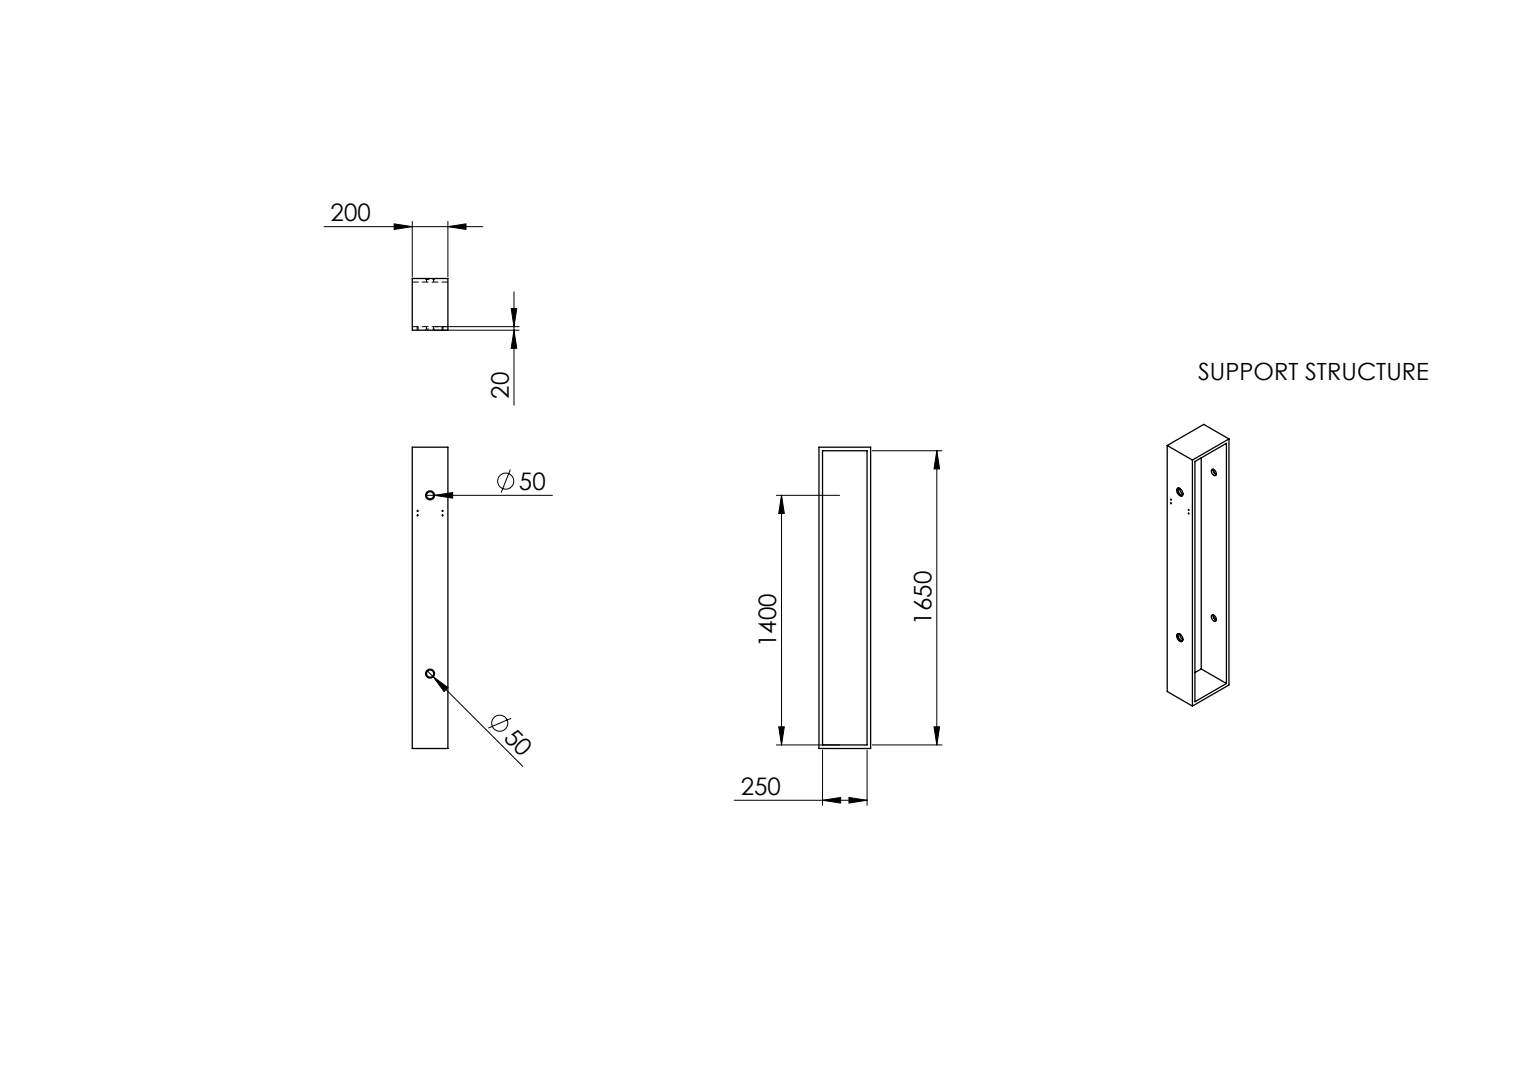
ISO-10303-21;
HEADER;
FILE_DESCRIPTION (('STEP AP214'),
    '1' );
FILE_NAME ('support structure.step',
    '2026-10-31T03:46:07',
    ( '' ),
    ( '' ),
    'SwSTEP 2.0',
    'SolidWorks 2026',
    '' );
FILE_SCHEMA (( 'AUTOMOTIVE_DESIGN' ));
ENDSEC;

DATA;
#3=VECTOR ( 'NONE', #6324, 1000.000000000000000 ) ;
#6=CARTESIAN_POINT ( 'NONE',  ( 18.83467029480910071, -16.52066876451827326, 145.0000119999999697 ) ) ;
#19=EDGE_CURVE ( 'NONE', #8380, #2021, #17168, .T. ) ;
#27=DIRECTION ( 'NONE',  ( 0.000000000000000000, 1.177509268541832635E-16, -1.000000000000000000 ) ) ;
#28=CARTESIAN_POINT ( 'NONE',  ( 15.24974479720505549, -1019.877690639539310, 145.0000119999999697 ) ) ;
#41=ORIENTED_EDGE ( 'NONE', *, *, #15976, .F. ) ;
#54=EDGE_LOOP ( 'NONE', ( #6384, #11170, #16002, #7000 ) ) ;
#58=DIRECTION ( 'NONE',  ( -1.000000000000000000, 0.000000000000000000, 0.000000000000000000 ) ) ;
#77=CARTESIAN_POINT ( 'NONE',  ( -69.99999999999997158, -87.33333333333338544, 145.0000000000000000 ) ) ;
#79=ORIENTED_EDGE ( 'NONE', *, *, #18426, .F. ) ;
#86=DIRECTION ( 'NONE',  ( 1.000000000000000000, 0.000000000000000000, 0.000000000000000000 ) ) ;
#96=CARTESIAN_POINT ( 'NONE',  ( 0.000000000000000000, -1000.000000000000000, 138.9999999999999716 ) ) ;
#102=CARTESIAN_POINT ( 'NONE',  ( 100.0000000000000000, 249.9999999999999716, 125.0000000000000284 ) ) ;
#108=LINE ( 'NONE', #2015, #19648 ) ;
#115=CARTESIAN_POINT ( 'NONE',  ( -11.07878015919984982, -22.47082401081930669, 145.0000119999999697 ) ) ;
#165=CIRCLE ( 'NONE', #9426, 5.249999999999949374 ) ;
#175=ORIENTED_EDGE ( 'NONE', *, *, #23587, .F. ) ;
#179=EDGE_CURVE ( 'NONE', #21239, #21516, #2397, .T. ) ;
#193=DIRECTION ( 'NONE',  ( 0.000000000000000000, 1.177509268541832635E-16, -1.000000000000000000 ) ) ;
#207=AXIS2_PLACEMENT_3D ( 'NONE', #19783, #10642, #8811 ) ;
#218=VERTEX_POINT ( 'NONE', #2274 ) ;
#224=DIRECTION ( 'NONE',  ( 0.000000000000000000, -1.000000000000000000, -1.177509268541832635E-16 ) ) ;
#245=EDGE_LOOP ( 'NONE', ( #12750, #13760, #3479, #23001 ) ) ;
#247=CYLINDRICAL_SURFACE ( 'NONE', #10836, 20.00000000000000000 ) ;
#257=ORIENTED_EDGE ( 'NONE', *, *, #4493, .F. ) ;
#312=DIRECTION ( 'NONE',  ( 0.000000000000000000, -1.000000000000000000, 0.000000000000000000 ) ) ;
#342=CARTESIAN_POINT ( 'NONE',  ( -24.99999999999998224, -1000.000000000000000, -145.0000119999999697 ) ) ;
#356=CARTESIAN_POINT ( 'NONE',  ( 21.69578997558840072, -12.52876685377503740, 145.0000119999999697 ) ) ;
#358=ADVANCED_FACE ( 'NONE', ( #20999 ), #19173, .F. ) ;
#362=PRODUCT_DEFINITION_CONTEXT ( 'detailed design', #17104, 'design' ) ;
#375=DIRECTION ( 'NONE',  ( -0.000000000000000000, 1.000000000000000000, -0.000000000000000000 ) ) ;
#385=CARTESIAN_POINT ( 'NONE',  ( 24.83884780301425721, -996.7275481119215783, 145.0000119999999981 ) ) ;
#391=ORIENTED_EDGE ( 'NONE', *, *, #9476, .F. ) ;
#411=ORIENTED_EDGE ( 'NONE', *, *, #12338, .T. ) ;
#419=DIRECTION ( 'NONE',  ( 0.000000000000000000, 1.177509268541832635E-16, -1.000000000000000000 ) ) ;
#431=EDGE_CURVE ( 'NONE', #23382, #2113, #16801, .T. ) ;
#434=LINE ( 'NONE', #15168, #15820 ) ;
#446=DIRECTION ( 'NONE',  ( 0.000000000000000000, -1.177509268541832635E-16, 1.000000000000000000 ) ) ;
#448=CARTESIAN_POINT ( 'NONE',  ( 70.00000000000000000, -87.33333333333332860, 124.9999999999999858 ) ) ;
#463=ADVANCED_FACE ( 'NONE', ( #11105 ), #20128, .F. ) ;
#476=DIRECTION ( 'NONE',  ( -0.000000000000000000, -0.000000000000000000, 1.000000000000000000 ) ) ;
#485=CARTESIAN_POINT ( 'NONE',  ( -45.00000000000000000, 272.9999999999999432, 0.000000000000000000 ) ) ;
#490=EDGE_CURVE ( 'NONE', #8328, #14713, #20594, .T. ) ;
#496=CARTESIAN_POINT ( 'NONE',  ( -24.99999999999998224, -1000.000000000000000, -145.0000060000000417 ) ) ;
#527=LINE ( 'NONE', #18858, #1845 ) ;
#529=ORIENTED_EDGE ( 'NONE', *, *, #11440, .F. ) ;
#546=CYLINDRICAL_SURFACE ( 'NONE', #5912, 20.00000000000000000 ) ;
#562=FACE_BOUND ( 'NONE', #6176, .T. ) ;
#563=DIRECTION ( 'NONE',  ( 0.000000000000000000, 0.000000000000000000, 1.000000000000000000 ) ) ;
#567=FACE_OUTER_BOUND ( 'NONE', #20459, .T. ) ;
#570=FACE_OUTER_BOUND ( 'NONE', #6214, .T. ) ;
#574=CARTESIAN_POINT ( 'NONE',  ( -69.99999999999997158, -112.6666666666667140, 124.9999999999999858 ) ) ;
#575=DIRECTION ( 'NONE',  ( 0.000000000000000000, 1.000000000000000000, 0.000000000000000000 ) ) ;
#576=ORIENTED_EDGE ( 'NONE', *, *, #2075, .T. ) ;
#589=CLOSED_SHELL ( 'NONE', ( #11368, #788, #23385, #20795, #2609, #21444, #6790, #9900, #8687, #7105, #11204, #10218, #16290, #19058, #463, #16239, #358, #10479, #18110, #9024, #1914, #5319, #16488, #1601, #20906, #2345, #19700, #11952, #5464, #626, #8870, #13898, #20498, #5716, #16281, #4561, #17901, #4387, #5710, #23652, #11628, #12501, #17871, #17586, #23607, #23039, #14935, #17741, #20750, #1436 ) ) ;
#612=CARTESIAN_POINT ( 'NONE',  ( -3.267023609986814847, -1024.839877336693462, -145.0000000000001421 ) ) ;
#615=CARTESIAN_POINT ( 'NONE',  ( 18.83467029480909005, -983.4793312354817090, 145.0000119999999697 ) ) ;
#626=ADVANCED_FACE ( 'NONE', ( #13405, #570 ), #13541, .T. ) ;
#637=DIRECTION ( 'NONE',  ( -0.000000000000000000, -0.000000000000000000, 1.000000000000000000 ) ) ;
#642=AXIS2_PLACEMENT_3D ( 'NONE', #1473, #5465, #8869 ) ;
#654=DIRECTION ( 'NONE',  ( 1.000000000000000000, 0.000000000000000000, 0.000000000000000000 ) ) ;
#657=DIRECTION ( 'NONE',  ( 0.000000000000000000, 1.177509268541832635E-16, -1.000000000000000000 ) ) ;
#665=ORIENTED_EDGE ( 'NONE', *, *, #13392, .T. ) ;
#670=LINE ( 'NONE', #6231, #14453 ) ;
#675=FACE_BOUND ( 'NONE', #20400, .T. ) ;
#691=DIRECTION ( 'NONE',  ( 0.000000000000000000, -1.177509268541832635E-16, 1.000000000000000000 ) ) ;
#702=CARTESIAN_POINT ( 'NONE',  ( -45.24999999999994316, 100.0000000000000000, -125.0000000000000000 ) ) ;
#710=CARTESIAN_POINT ( 'NONE',  ( -24.99999999999998224, -1000.000000000000000, 145.0000119999999697 ) ) ;
#719=AXIS2_PLACEMENT_3D ( 'NONE', #14243, #1403, #19754 ) ;
#735=STYLED_ITEM('',(#23934),#20017);
#755=CARTESIAN_POINT ( 'NONE',  ( -16.51661848988935688, -981.1612097654584659, -145.0000000000001137 ) ) ;
#777=CARTESIAN_POINT ( 'NONE',  ( 67.35000000000002274, -112.6666666666666714, 148.0000000000000000 ) ) ;
#788=ADVANCED_FACE ( 'NONE', ( #20967 ), #6715, .F. ) ;
#791=CARTESIAN_POINT ( 'NONE',  ( -15.25452100743371275, 19.87444003246448077, -145.0000000000000000 ) ) ;
#798=CYLINDRICAL_SURFACE ( 'NONE', #13137, 20.00000000000000000 ) ;
#815=DIRECTION ( 'NONE',  ( -1.000000000000000000, -0.000000000000000000, -0.000000000000000000 ) ) ;
#853=CARTESIAN_POINT ( 'NONE',  ( 16.51667796972429514, -18.83873075115305440, -145.0000000000000000 ) ) ;
#864=CARTESIAN_POINT ( 'NONE',  ( -24.19933745276217252, -993.5122599704404820, -145.0000000000001137 ) ) ;
#883=FACE_BOUND ( 'NONE', #18234, .T. ) ;
#888=CYLINDRICAL_SURFACE ( 'NONE', #2282, 20.00000000000000000 ) ;
#891=CARTESIAN_POINT ( 'NONE',  ( -21.69892645963121325, 12.52401366518118841, -145.0000000000000000 ) ) ;
#903=ORIENTED_EDGE ( 'NONE', *, *, #3665, .F. ) ;
#916=FACE_BOUND ( 'NONE', #6482, .T. ) ;
#917=DIRECTION ( 'NONE',  ( 1.000000000000000000, 0.000000000000000000, 0.000000000000000000 ) ) ;
#926=CARTESIAN_POINT ( 'NONE',  ( 0.000000000000000000, 0.000000000000000000, 138.9999999999999716 ) ) ;
#930=CIRCLE ( 'NONE', #16749, 5.249999999999949374 ) ;
#940=EDGE_CURVE ( 'NONE', #17429, #3770, #2550, .T. ) ;
#948=CYLINDRICAL_SURFACE ( 'NONE', #18630, 2.649999999999985700 ) ;
#954=DIRECTION ( 'NONE',  ( -1.000000000000000000, -0.000000000000000000, -0.000000000000000000 ) ) ;
#965=CARTESIAN_POINT ( 'NONE',  ( -23.72540896994113524, -8.050072860292576848, -145.0000000000000000 ) ) ;
#975=CARTESIAN_POINT ( 'NONE',  ( -1.642023387942652235, -975.0000492607058504, -145.0000000000001421 ) ) ;
#981=SURFACE_STYLE_USAGE ( .BOTH. , #17532 ) ;
#997=B_SPLINE_CURVE_WITH_KNOTS ( 'NONE', 3,
 ( #16561, #14521, #9199, #21855, #11385, #5449, #16437, #14640, #23787, #12745, #3867, #5814, #18479, #16679, #5326, #16789, #14756, #7484, #18699, #20277, #9325, #7604, #12857, #28, #20057, #10914, #18236, #9077, #14997, #13218, #20519, #22087, #3732, #7245 ),
 .UNSPECIFIED., .F., .F.,
 ( 4, 2, 2, 2, 2, 2, 2, 2, 2, 2, 2, 2, 2, 2, 2, 2, 4 ),
 ( 0.5000000000000000000, 0.5312500000000000000, 0.5625000000000000000, 0.5937500000000000000, 0.6250000000000000000, 0.6562500000000000000, 0.6875000000000000000, 0.7187500000000000000, 0.7500000000000000000, 0.7812500000000000000, 0.8125000000000000000, 0.8437500000000000000, 0.8750000000000000000, 0.9062500000000000000, 0.9375000000000000000, 0.9687500000000000000, 1.000000000000000000 ),
 .UNSPECIFIED. ) ;
#1003=DIRECTION ( 'NONE',  ( 0.000000000000000000, 1.000000000000000000, 0.000000000000000000 ) ) ;
#1007=CARTESIAN_POINT ( 'NONE',  ( 6.487740029101478179, 24.19933745276211212, -145.0000000000000000 ) ) ;
#1022=CYLINDRICAL_SURFACE ( 'NONE', #9203, 25.00000000000000000 ) ;
#1068=FACE_OUTER_BOUND ( 'NONE', #19426, .T. ) ;
#1088=CARTESIAN_POINT ( 'NONE',  ( 12.52399064345484980, -21.69904058272398117, -145.0000000000000000 ) ) ;
#1106=ORIENTED_EDGE ( 'NONE', *, *, #5078, .F. ) ;
#1142=CIRCLE ( 'NONE', #20035, 2.649999999999999467 ) ;
#1161=STYLED_ITEM ( 'NONE', ( #8363 ), #19351 ) ;
#1173=EDGE_LOOP ( 'NONE', ( #15595, #19148, #21434, #576 ) ) ;
#1179=CYLINDRICAL_SURFACE ( 'NONE', #16892, 5.249999999999973355 ) ;
#1187=CARTESIAN_POINT ( 'NONE',  ( 67.35000000000002274, -87.33333333333332860, 124.9999999999999858 ) ) ;
#1198=LINE ( 'NONE', #13923, #16019 ) ;
#1200=ORIENTED_EDGE ( 'NONE', *, *, #4425, .F. ) ;
#1202=DIRECTION ( 'NONE',  ( 1.000000000000000000, 0.000000000000000000, 0.000000000000000000 ) ) ;
#1254=ORIENTED_EDGE ( 'NONE', *, *, #16181, .T. ) ;
#1279=CARTESIAN_POINT ( 'NONE',  ( 45.24999999999994316, 100.0000000000000000, 150.2000000000009550 ) ) ;
#1288=CARTESIAN_POINT ( 'NONE',  ( -20.00000000000000000, 2.449293598294706513E-15, -125.0000000000000000 ) ) ;
#1294=CARTESIAN_POINT ( 'NONE',  ( -20.00000000000000000, -1000.000000000000000, 124.9999999999998579 ) ) ;
#1302=DIRECTION ( 'NONE',  ( 0.000000000000000000, 0.000000000000000000, -1.000000000000000000 ) ) ;
#1314=VERTEX_POINT ( 'NONE', #2400 ) ;
#1326=DIRECTION ( 'NONE',  ( 0.000000000000000000, 1.177509268541832635E-16, -1.000000000000000000 ) ) ;
#1339=CYLINDRICAL_SURFACE ( 'NONE', #13540, 24.99999999999998224 ) ;
#1390=DIRECTION ( 'NONE',  ( 0.000000000000000000, 1.177509268541832635E-16, -1.000000000000000000 ) ) ;
#1394=DIRECTION ( 'NONE',  ( -0.000000000000000000, -0.000000000000000000, 1.000000000000000000 ) ) ;
#1403=DIRECTION ( 'NONE',  ( -0.000000000000000000, -1.177509268541832635E-16, 1.000000000000000000 ) ) ;
#1436=ADVANCED_FACE ( 'NONE', ( #13210 ), #20510, .F. ) ;
#1454=DIRECTION ( 'NONE',  ( -1.000000000000000000, 0.000000000000000000, 0.000000000000000000 ) ) ;
#1466=ORIENTED_EDGE ( 'NONE', *, *, #21900, .T. ) ;
#1472=EDGE_CURVE ( 'NONE', #15247, #5237, #1198, .T. ) ;
#1473=CARTESIAN_POINT ( 'NONE',  ( -40.00000000000000000, 100.0000000000000000, 145.0000000000000000 ) ) ;
#1487=VERTEX_POINT ( 'NONE', #8213 ) ;
#1500=VECTOR ( 'NONE', #17474, 1000.000000000000000 ) ;
#1504=CIRCLE ( 'NONE', #2664, 5.249999999999949374 ) ;
#1521=VECTOR ( 'NONE', #15755, 1000.000000000000000 ) ;
#1535=CARTESIAN_POINT ( 'NONE',  ( 6.482064212728078090, 24.20041621714725721, 145.0000119999999697 ) ) ;
#1558=DIRECTION ( 'NONE',  ( 0.000000000000000000, -1.110223024625156540E-16, 1.000000000000000000 ) ) ;
#1572=CARTESIAN_POINT ( 'NONE',  ( 6.482064212728086972, -24.20041621714725011, 145.0000119999999697 ) ) ;
#1578=EDGE_LOOP ( 'NONE', ( #14590, #13725 ) ) ;
#1586=EDGE_CURVE ( 'NONE', #12471, #4961, #8307, .T. ) ;
#1597=ORIENTED_EDGE ( 'NONE', *, *, #13231, .F. ) ;
#1601=ADVANCED_FACE ( 'NONE', ( #9043 ), #3478, .F. ) ;
#1624=CIRCLE ( 'NONE', #13627, 2.649999999999985700 ) ;
#1628=ORIENTED_EDGE ( 'NONE', *, *, #5078, .T. ) ;
#1650=CARTESIAN_POINT ( 'NONE',  ( 0.000000000000000000, 1.865214261513747767E-15, 145.0000119999999697 ) ) ;
#1656=ORIENTED_EDGE ( 'NONE', *, *, #2894, .T. ) ;
#1668=ORIENTED_EDGE ( 'NONE', *, *, #13168, .T. ) ;
#1687=PRODUCT ( 'support structure', 'support structure', '', ( #5653 ) ) ;
#1700=ORIENTED_EDGE ( 'NONE', *, *, #10708, .F. ) ;
#1705=ORIENTED_EDGE ( 'NONE', *, *, #18577, .F. ) ;
#1736=DIRECTION ( 'NONE',  ( -0.000000000000000000, -0.000000000000000000, 1.000000000000000000 ) ) ;
#1788=CARTESIAN_POINT ( 'NONE',  ( -12.52876685377503385, -21.69578997558839717, 145.0000119999999981 ) ) ;
#1809=DIRECTION ( 'NONE',  ( 0.000000000000000000, 0.000000000000000000, 1.000000000000000000 ) ) ;
#1811=LINE ( 'NONE', #9206, #10408 ) ;
#1823=FACE_OUTER_BOUND ( 'NONE', #12229, .T. ) ;
#1825=EDGE_CURVE ( 'NONE', #13236, #17386, #21895, .T. ) ;
#1845=VECTOR ( 'NONE', #954, 1000.000000000000000 ) ;
#1872=FACE_OUTER_BOUND ( 'NONE', #23417, .T. ) ;
#1889=EDGE_LOOP ( 'NONE', ( #14035, #13919, #9509, #20790 ) ) ;
#1907=DIRECTION ( 'NONE',  ( -0.000000000000000000, -0.000000000000000000, 1.000000000000000000 ) ) ;
#1912=ORIENTED_EDGE ( 'NONE', *, *, #7800, .F. ) ;
#1914=ADVANCED_FACE ( 'NONE', ( #17471, #916 ), #21219, .T. ) ;
#1956=VERTEX_POINT ( 'NONE', #10856 ) ;
#1957=DIRECTION ( 'NONE',  ( -0.000000000000000000, -0.000000000000000000, 1.000000000000000000 ) ) ;
#1967=DIRECTION ( 'NONE',  ( 0.000000000000000000, 1.000000000000000000, 0.000000000000000000 ) ) ;
#1991=DIRECTION ( 'NONE',  ( -0.000000000000000000, -0.000000000000000000, 1.000000000000000000 ) ) ;
#2002=EDGE_CURVE ( 'NONE', #18582, #6504, #3774, .T. ) ;
#2006=ORIENTED_EDGE ( 'NONE', *, *, #20259, .F. ) ;
#2015=CARTESIAN_POINT ( 'NONE',  ( 100.0000000000000000, 249.9999999999999716, 125.0000000000000284 ) ) ;
#2019=CARTESIAN_POINT ( 'NONE',  ( -40.00000000000000000, 100.0000000000000000, 125.0000000000000000 ) ) ;
#2020=EDGE_LOOP ( 'NONE', ( #17265, #10424, #23573, #20503 ) ) ;
#2021=VERTEX_POINT ( 'NONE', #18282 ) ;
#2023=EDGE_CURVE ( 'NONE', #16783, #7859, #14353, .T. ) ;
#2043=DIRECTION ( 'NONE',  ( -0.000000000000000000, -0.000000000000000000, 1.000000000000000000 ) ) ;
#2050=( NAMED_UNIT ( * ) SI_UNIT ( $, .STERADIAN. ) SOLID_ANGLE_UNIT ( ) );
#2061=EDGE_CURVE ( 'NONE', #23382, #13229, #21904, .T. ) ;
#2067=DIRECTION ( 'NONE',  ( 1.000000000000000000, 0.000000000000000000, 0.000000000000000000 ) ) ;
#2069=VERTEX_POINT ( 'NONE', #18627 ) ;
#2075=EDGE_CURVE ( 'NONE', #21835, #17715, #16831, .T. ) ;
#2082=CARTESIAN_POINT ( 'NONE',  ( 24.99999999999998224, -1000.000000000000000, 138.9999999999999716 ) ) ;
#2096=CARTESIAN_POINT ( 'NONE',  ( -6.482064212728105623, -975.7995837828526646, 145.0000119999999697 ) ) ;
#2101=EDGE_CURVE ( 'NONE', #2069, #12336, #14538, .T. ) ;
#2113=VERTEX_POINT ( 'NONE', #5610 ) ;
#2118=VERTEX_POINT ( 'NONE', #22257 ) ;
#2120=CYLINDRICAL_SURFACE ( 'NONE', #2712, 20.00000000000000000 ) ;
#2139=ORIENTED_EDGE ( 'NONE', *, *, #12338, .F. ) ;
#2148=DIRECTION ( 'NONE',  ( -0.000000000000000000, 1.000000000000000000, -0.000000000000000000 ) ) ;
#2151=AXIS2_PLACEMENT_3D ( 'NONE', #13145, #20452, #18988 ) ;
#2183=AXIS2_PLACEMENT_3D ( 'NONE', #6288, #21018, #15246 ) ;
#2192=DIRECTION ( 'NONE',  ( 0.000000000000000000, 1.177509268541832635E-16, -1.000000000000000000 ) ) ;
#2214=CARTESIAN_POINT ( 'NONE',  ( -3.272451888078324433, -975.1611521969856540, 145.0000119999999697 ) ) ;
#2232=AXIS2_PLACEMENT_3D ( 'NONE', #15906, #3082, #23243 ) ;
#2260=ORIENTED_EDGE ( 'NONE', *, *, #16101, .T. ) ;
#2263=AXIS2_PLACEMENT_3D ( 'NONE', #3156, #11909, #19217 ) ;
#2270=EDGE_CURVE ( 'NONE', #15596, #21835, #19465, .T. ) ;
#2274=CARTESIAN_POINT ( 'NONE',  ( -25.00000000000000000, 1.865214261513747767E-15, -138.9999999999999716 ) ) ;
#2282=AXIS2_PLACEMENT_3D ( 'NONE', #9976, #11933, #2927 ) ;
#2284=CARTESIAN_POINT ( 'NONE',  ( 72.64999999999999147, -87.33333333333332860, 145.0000000000000000 ) ) ;
#2290=CARTESIAN_POINT ( 'NONE',  ( -34.75000000000005684, 100.0000000000000000, -125.0000000000000000 ) ) ;
#2324=CARTESIAN_POINT ( 'NONE',  ( -24.99999999999998224, -1000.000000000000000, -145.0000060000000417 ) ) ;
#2326=VECTOR ( 'NONE', #14074, 1000.000000000000000 ) ;
#2332=ORIENTED_EDGE ( 'NONE', *, *, #9667, .F. ) ;
#2335=CARTESIAN_POINT ( 'NONE',  ( 45.24999999999994316, 100.0000000000000000, 125.0000000000000000 ) ) ;
#2340=VERTEX_POINT ( 'NONE', #17443 ) ;
#2345=ADVANCED_FACE ( 'NONE', ( #883, #8262, #2577 ), #9970, .T. ) ;
#2367=ORIENTED_EDGE ( 'NONE', *, *, #2518, .F. ) ;
#2393=EDGE_LOOP ( 'NONE', ( #11641, #12163, #21345, #5733 ) ) ;
#2397=LINE ( 'NONE', #6023, #2469 ) ;
#2400=CARTESIAN_POINT ( 'NONE',  ( -45.24999999999994316, 100.0000000000000000, 125.0000000000000000 ) ) ;
#2410=CARTESIAN_POINT ( 'NONE',  ( -15.25457574233255365, -1019.874521950566759, -145.0000000000001137 ) ) ;
#2430=AXIS2_PLACEMENT_3D ( 'NONE', #2688, #637, #10084 ) ;
#2454=LINE ( 'NONE', #4392, #6464 ) ;
#2467=CARTESIAN_POINT ( 'NONE',  ( -19.87455415549606741, 15.25449798579914251, -145.0000000000000000 ) ) ;
#2469=VECTOR ( 'NONE', #9783, 1000.000000000000000 ) ;
#2472=EDGE_CURVE ( 'NONE', #22877, #18582, #8983, .T. ) ;
#2482=FACE_BOUND ( 'NONE', #3832, .T. ) ;
#2491=DIRECTION ( 'NONE',  ( 1.000000000000000000, 0.000000000000000000, -0.000000000000000000 ) ) ;
#2518=EDGE_CURVE ( 'NONE', #12660, #5442, #23460, .T. ) ;
#2524=ORIENTED_EDGE ( 'NONE', *, *, #15478, .T. ) ;
#2525=CARTESIAN_POINT ( 'NONE',  ( 100.0000000000000000, 270.0000000000000000, -144.9999999999999716 ) ) ;
#2532=AXIS2_PLACEMENT_3D ( 'NONE', #17832, #23249, #10011 ) ;
#2538=CARTESIAN_POINT ( 'NONE',  ( -34.75000000000005684, 100.0000000000000000, -145.0000000000000284 ) ) ;
#2550=LINE ( 'NONE', #13707, #11792 ) ;
#2574=DIRECTION ( 'NONE',  ( 0.000000000000000000, 0.000000000000000000, 1.000000000000000000 ) ) ;
#2577=FACE_OUTER_BOUND ( 'NONE', #18376, .T. ) ;
#2580=FACE_OUTER_BOUND ( 'NONE', #2393, .T. ) ;
#2582=FACE_OUTER_BOUND ( 'NONE', #245, .T. ) ;
#2587=CARTESIAN_POINT ( 'NONE',  ( -100.0000000000000000, -1420.000000000000000, -145.0000000000001705 ) ) ;
#2609=ADVANCED_FACE ( 'NONE', ( #11298 ), #16589, .F. ) ;
#2632=AXIS2_PLACEMENT_3D ( 'NONE', #12238, #7885, #20671 ) ;
#2664=AXIS2_PLACEMENT_3D ( 'NONE', #12447, #16140, #4785 ) ;
#2666=ORIENTED_EDGE ( 'NONE', *, *, #16101, .F. ) ;
#2669=CARTESIAN_POINT ( 'NONE',  ( 11.08409875733031136, -22.46856765614143825, -145.0000000000000000 ) ) ;
#2674=CIRCLE ( 'NONE', #13520, 2.649999999999999467 ) ;
#2683=EDGE_CURVE ( 'NONE', #15535, #5442, #9705, .T. ) ;
#2688=CARTESIAN_POINT ( 'NONE',  ( 70.00000000000000000, -87.33333333333332860, 148.0000000000000000 ) ) ;
#2712=AXIS2_PLACEMENT_3D ( 'NONE', #11711, #20855, #4176 ) ;
#2715=AXIS2_PLACEMENT_3D ( 'NONE', #22993, #6348, #10119 ) ;
#2718=CARTESIAN_POINT ( 'NONE',  ( 0.000000000000000000, 0.000000000000000000, 124.9999999999999716 ) ) ;
#2728=DIRECTION ( 'NONE',  ( 1.000000000000000000, 0.000000000000000000, 0.000000000000000000 ) ) ;
#2735=EDGE_LOOP ( 'NONE', ( #4395, #3923 ) ) ;
#2746=CARTESIAN_POINT ( 'NONE',  ( -100.0000000000000000, -1420.000000000000000, 144.9999999999998295 ) ) ;
#2763=ORIENTED_EDGE ( 'NONE', *, *, #22787, .F. ) ;
#2783=CARTESIAN_POINT ( 'NONE',  ( 23.72528575883189816, -8.050112875864174455, -145.0000000000000000 ) ) ;
#2786=PLANE ( 'NONE',  #17177 ) ;
#2807=CARTESIAN_POINT ( 'NONE',  ( 45.00000000000000000, 272.9999999999999432, -5.249999999999973355 ) ) ;
#2822=CARTESIAN_POINT ( 'NONE',  ( -24.19933745025247873, 6.487655866515821046, -145.0000000000000000 ) ) ;
#2832=DIRECTION ( 'NONE',  ( 0.000000000000000000, 1.177509268541832635E-16, -1.000000000000000000 ) ) ;
#2835=CYLINDRICAL_SURFACE ( 'NONE', #4202, 24.99999999999998224 ) ;
#2851=CARTESIAN_POINT ( 'NONE',  ( -18.83879023463319058, -1016.516618489828488, -145.0000000000001421 ) ) ;
#2861=AXIS2_PLACEMENT_3D ( 'NONE', #5285, #3576, #3224 ) ;
#2869=FACE_BOUND ( 'NONE', #4565, .T. ) ;
#2875=AXIS2_PLACEMENT_3D ( 'NONE', #4426, #11837, #21216 ) ;
#2879=ORIENTED_EDGE ( 'NONE', *, *, #13422, .F. ) ;
#2886=CARTESIAN_POINT ( 'NONE',  ( -21.69904058246457268, -12.52399064369876669, -145.0000000000000000 ) ) ;
#2894=EDGE_CURVE ( 'NONE', #4083, #13410, #9654, .T. ) ;
#2921=CARTESIAN_POINT ( 'NONE',  ( 20.00000000000000000, -1000.000000000000000, -150.0000000000000000 ) ) ;
#2927=DIRECTION ( 'NONE',  ( 1.000000000000000000, 0.000000000000000000, 0.000000000000000000 ) ) ;
#2934=EDGE_CURVE ( 'NONE', #21516, #7464, #17374, .T. ) ;
#2949=DIRECTION ( 'NONE',  ( 0.000000000000000000, 1.000000000000000000, 0.000000000000000000 ) ) ;
#2989=VERTEX_POINT ( 'NONE', #20978 ) ;
#3011=CARTESIAN_POINT ( 'NONE',  ( -15.25450579711302623, -19.87456868343288363, -145.0000000000000000 ) ) ;
#3014=FACE_BOUND ( 'NONE', #15228, .T. ) ;
#3040=CIRCLE ( 'NONE', #12737, 25.00000000000000000 ) ;
#3053=CARTESIAN_POINT ( 'NONE',  ( 100.0000000000000000, 249.9999999999999716, 125.0000000000000284 ) ) ;
#3082=DIRECTION ( 'NONE',  ( -0.000000000000000000, -0.000000000000000000, 1.000000000000000000 ) ) ;
#3084=VECTOR ( 'NONE', #7877, 1000.000000000000000 ) ;
#3094=VERTEX_POINT ( 'NONE', #2746 ) ;
#3100=CARTESIAN_POINT ( 'NONE',  ( -34.75000000000005684, 100.0000000000000000, 125.0000000000000000 ) ) ;
#3104=LINE ( 'NONE', #3480, #11493 ) ;
#3111=CARTESIAN_POINT ( 'NONE',  ( 0.000000000000000000, -1000.000000000000000, 124.9999999999998579 ) ) ;
#3119=EDGE_CURVE ( 'NONE', #3718, #13209, #8415, .T. ) ;
#3144=ORIENTED_EDGE ( 'NONE', *, *, #2061, .F. ) ;
#3156=CARTESIAN_POINT ( 'NONE',  ( 40.00000000000000000, 100.0000000000000000, 150.2000000000009550 ) ) ;
#3170=ORIENTED_EDGE ( 'NONE', *, *, #14229, .F. ) ;
#3179=CARTESIAN_POINT ( 'NONE',  ( 0.000000000000000000, 0.000000000000000000, -125.0000000000000000 ) ) ;
#3202=EDGE_CURVE ( 'NONE', #2989, #7088, #11950, .T. ) ;
#3212=ORIENTED_EDGE ( 'NONE', *, *, #2061, .T. ) ;
#3224=DIRECTION ( 'NONE',  ( -1.000000000000000000, 0.000000000000000000, 0.000000000000000000 ) ) ;
#3263=CARTESIAN_POINT ( 'NONE',  ( 0.000000000000000000, -1000.000000000000000, 145.0000119999999697 ) ) ;
#3270=CARTESIAN_POINT ( 'NONE',  ( 20.00000000000000000, 0.000000000000000000, -125.0000000000000000 ) ) ;
#3278=CARTESIAN_POINT ( 'NONE',  ( -45.00000000000000000, 272.9999999999999432, 5.249999999999973355 ) ) ;
#3282=DIRECTION ( 'NONE',  ( 1.000000000000000000, 0.000000000000000000, 0.000000000000000000 ) ) ;
#3301=AXIS2_PLACEMENT_3D ( 'NONE', #6837, #13774, #21092 ) ;
#3323=VECTOR ( 'NONE', #5730, 1000.000000000000000 ) ;
#3347=VERTEX_POINT ( 'NONE', #4994 ) ;
#3351=ORIENTED_EDGE ( 'NONE', *, *, #3665, .T. ) ;
#3352=LINE ( 'NONE', #102, #22254 ) ;
#3391=EDGE_LOOP ( 'NONE', ( #6494, #9496, #6292, #22641 ) ) ;
#3397=DIRECTION ( 'NONE',  ( 0.000000000000000000, -1.000000000000000000, 0.000000000000000000 ) ) ;
#3434=EDGE_CURVE ( 'NONE', #15247, #20600, #1504, .T. ) ;
#3461=CARTESIAN_POINT ( 'NONE',  ( -12.52876685377504451, 21.69578997558840072, 145.0000119999999697 ) ) ;
#3477=ORIENTED_EDGE ( 'NONE', *, *, #21259, .T. ) ;
#3478=PLANE ( 'NONE',  #21787 ) ;
#3479=ORIENTED_EDGE ( 'NONE', *, *, #2101, .T. ) ;
#3480=CARTESIAN_POINT ( 'NONE',  ( -45.24999999999994316, 100.0000000000000000, 150.2000000000009550 ) ) ;
#3494=CARTESIAN_POINT ( 'NONE',  ( -22.47082401081931735, -11.07878015919985515, 145.0000119999999697 ) ) ;
#3522=DIRECTION ( 'NONE',  ( -0.000000000000000000, -0.000000000000000000, 1.000000000000000000 ) ) ;
#3564=CARTESIAN_POINT ( 'NONE',  ( -22.47082401081932090, 11.07878015919984804, 145.0000119999999697 ) ) ;
#3576=DIRECTION ( 'NONE',  ( 0.000000000000000000, 0.000000000000000000, 1.000000000000000000 ) ) ;
#3612=CARTESIAN_POINT ( 'NONE',  ( 0.000000000000000000, 1.865214261513747767E-15, 138.9999999999999716 ) ) ;
#3640=ORIENTED_EDGE ( 'NONE', *, *, #8742, .F. ) ;
#3641=CARTESIAN_POINT ( 'NONE',  ( 12.52393590769071174, -978.3010413347997201, -145.0000000000001421 ) ) ;
#3645=DIRECTION ( 'NONE',  ( -0.000000000000000000, -0.000000000000000000, 1.000000000000000000 ) ) ;
#3651=CIRCLE ( 'NONE', #18698, 24.99999999999998224 ) ;
#3662=EDGE_CURVE ( 'NONE', #14636, #13229, #1142, .T. ) ;
#3663=EDGE_LOOP ( 'NONE', ( #16770, #8204 ) ) ;
#3665=EDGE_CURVE ( 'NONE', #13236, #2021, #20937, .T. ) ;
#3698=ORIENTED_EDGE ( 'NONE', *, *, #4824, .F. ) ;
#3703=ORIENTED_EDGE ( 'NONE', *, *, #8396, .F. ) ;
#3711=CYLINDRICAL_SURFACE ( 'NONE', #16171, 5.249999999999942268 ) ;
#3718=VERTEX_POINT ( 'NONE', #16971 ) ;
#3725=EDGE_CURVE ( 'NONE', #19888, #17037, #434, .T. ) ;
#3730=LINE ( 'NONE', #7483, #8110 ) ;
#3732=CARTESIAN_POINT ( 'NONE',  ( 24.99999999999998224, -1001.636246173744667, 145.0000119999999697 ) ) ;
#3750=CARTESIAN_POINT ( 'NONE',  ( -72.64999999999996305, -112.6666666666667140, 124.9999999999999858 ) ) ;
#3753=DIRECTION ( 'NONE',  ( 0.000000000000000000, 0.000000000000000000, -1.000000000000000000 ) ) ;
#3769=DIRECTION ( 'NONE',  ( 1.000000000000000000, 0.000000000000000000, 0.000000000000000000 ) ) ;
#3770=VERTEX_POINT ( 'NONE', #19840 ) ;
#3774=CIRCLE ( 'NONE', #10295, 24.99999999999998224 ) ;
#3778=AXIS2_PLACEMENT_3D ( 'NONE', #10990, #18309, #7338 ) ;
#3780=DIRECTION ( 'NONE',  ( 0.000000000000000000, 0.000000000000000000, 1.000000000000000000 ) ) ;
#3802=EDGE_CURVE ( 'NONE', #4083, #11935, #4647, .T. ) ;
#3810=ORIENTED_EDGE ( 'NONE', *, *, #18462, .T. ) ;
#3832=EDGE_LOOP ( 'NONE', ( #9105, #6349 ) ) ;
#3848=EDGE_CURVE ( 'NONE', #20062, #21409, #8378, .T. ) ;
#3867=CARTESIAN_POINT ( 'NONE',  ( -15.24974479720505371, -1019.877690639539082, 145.0000119999999697 ) ) ;
#3911=EDGE_LOOP ( 'NONE', ( #13777, #1597 ) ) ;
#3923=ORIENTED_EDGE ( 'NONE', *, *, #16663, .T. ) ;
#3929=AXIS2_PLACEMENT_3D ( 'NONE', #16439, #14643, #15000 ) ;
#3932=DIRECTION ( 'NONE',  ( -1.000000000000000000, -0.000000000000000000, -0.000000000000000000 ) ) ;
#3978=DIRECTION ( 'NONE',  ( 0.000000000000000000, 0.000000000000000000, -1.000000000000000000 ) ) ;
#4010=AXIS2_PLACEMENT_3D ( 'NONE', #5172, #9286, #20011 ) ;
#4044=DIRECTION ( 'NONE',  ( -0.000000000000000000, -0.000000000000000000, 1.000000000000000000 ) ) ;
#4072=ORIENTED_EDGE ( 'NONE', *, *, #2683, .F. ) ;
#4083=VERTEX_POINT ( 'NONE', #19558 ) ;
#4085=CARTESIAN_POINT ( 'NONE',  ( 100.0000000000000000, -1400.000000000000000, -145.0000000000001705 ) ) ;
#4091=AXIS2_PLACEMENT_3D ( 'NONE', #15289, #22620, #11433 ) ;
#4092=DIRECTION ( 'NONE',  ( -0.000000000000000000, 1.000000000000000000, -0.000000000000000000 ) ) ;
#4103=EDGE_LOOP ( 'NONE', ( #8311, #3351, #19843, #1700 ) ) ;
#4134=LINE ( 'NONE', #9362, #11637 ) ;
#4164=AXIS2_PLACEMENT_3D ( 'NONE', #18353, #12621, #17891 ) ;
#4176=DIRECTION ( 'NONE',  ( 1.000000000000000000, 0.000000000000000000, 0.000000000000000000 ) ) ;
#4181=EDGE_CURVE ( 'NONE', #21516, #13307, #8239, .T. ) ;
#4187=VECTOR ( 'NONE', #3645, 1000.000000000000000 ) ;
#4202=AXIS2_PLACEMENT_3D ( 'NONE', #12311, #15784, #10231 ) ;
#4203=CARTESIAN_POINT ( 'NONE',  ( 23.72315261474502890, -8.055391459054607850, 145.0000119999999697 ) ) ;
#4221=EDGE_LOOP ( 'NONE', ( #20755, #16672, #22624, #2139 ) ) ;
#4237=PRODUCT_DEFINITION_FORMATION_WITH_SPECIFIED_SOURCE ( 'ANY', '', #1687, .NOT_KNOWN. ) ;
#4261=FACE_OUTER_BOUND ( 'NONE', #6331, .T. ) ;
#4291=CARTESIAN_POINT ( 'NONE',  ( 12.52393590864757478, 21.69895866456091582, -145.0000000000000000 ) ) ;
#4332=EDGE_CURVE ( 'NONE', #20600, #5249, #7129, .T. ) ;
#4333=CARTESIAN_POINT ( 'NONE',  ( 24.99999999999999289, -1.636246173744675625, 145.0000119999999697 ) ) ;
#4348=DIRECTION ( 'NONE',  ( 1.000000000000000000, 0.000000000000000000, 0.000000000000000000 ) ) ;
#4362=CARTESIAN_POINT ( 'NONE',  ( -8.050117706004019880, -23.72530153055896207, -145.0000000000000000 ) ) ;
#4366=ORIENTED_EDGE ( 'NONE', *, *, #14229, .T. ) ;
#4372=UNCERTAINTY_MEASURE_WITH_UNIT (LENGTH_MEASURE( 1.000000000000000082E-05 ), #12426, 'distance_accuracy_value', 'NONE');
#4374=CYLINDRICAL_SURFACE ( 'NONE', #2430, 2.649999999999985700 ) ;
#4378=ORIENTED_EDGE ( 'NONE', *, *, #17960, .F. ) ;
#4387=ADVANCED_FACE ( 'NONE', ( #21746 ), #23783, .F. ) ;
#4392=CARTESIAN_POINT ( 'NONE',  ( 20.00000000000000000, 0.000000000000000000, -150.0000000000000000 ) ) ;
#4395=ORIENTED_EDGE ( 'NONE', *, *, #490, .T. ) ;
#4401=DIRECTION ( 'NONE',  ( 1.000000000000000000, 0.000000000000000000, 0.000000000000000000 ) ) ;
#4403=CARTESIAN_POINT ( 'NONE',  ( -16.51667796985407932, 18.83873075099288386, -145.0000000000000000 ) ) ;
#4411=DIRECTION ( 'NONE',  ( 0.000000000000000000, 1.000000000000000000, 0.000000000000000000 ) ) ;
#4420=VERTEX_POINT ( 'NONE', #2284 ) ;
#4425=EDGE_CURVE ( 'NONE', #21239, #17037, #9682, .T. ) ;
#4426=CARTESIAN_POINT ( 'NONE',  ( 45.00000000000000000, 272.9999999999999432, 0.000000000000000000 ) ) ;
#4435=DIRECTION ( 'NONE',  ( 1.000000000000000000, 0.000000000000000000, 0.000000000000000000 ) ) ;
#4438=FACE_OUTER_BOUND ( 'NONE', #13083, .T. ) ;
#4448=ORIENTED_EDGE ( 'NONE', *, *, #16677, .F. ) ;
#4468=DIRECTION ( 'NONE',  ( 0.000000000000000000, -1.000000000000000000, -1.177509268541832635E-16 ) ) ;
#4484=CARTESIAN_POINT ( 'NONE',  ( 6.487720807569985482, -24.19924082479899852, -145.0000000000000000 ) ) ;
#4493=EDGE_CURVE ( 'NONE', #13307, #7122, #13800, .T. ) ;
#4494=ORIENTED_EDGE ( 'NONE', *, *, #4824, .T. ) ;
#4496=CARTESIAN_POINT ( 'NONE',  ( 34.75000000000005684, 100.0000000000000000, 145.0000000000000000 ) ) ;
#4497=CARTESIAN_POINT ( 'NONE',  ( -11.08409875828705893, -977.5314323444980573, -145.0000000000001421 ) ) ;
#4509=DIRECTION ( 'NONE',  ( -0.000000000000000000, 1.000000000000000000, -0.000000000000000000 ) ) ;
#4512=DIRECTION ( 'NONE',  ( 1.000000000000000000, 0.000000000000000000, 0.000000000000000000 ) ) ;
#4523=DIRECTION ( 'NONE',  ( 0.000000000000000000, 1.000000000000000000, 0.000000000000000000 ) ) ;
#4525=CARTESIAN_POINT ( 'NONE',  ( 24.99999999999998224, -1000.000000000000000, 145.0000059999999280 ) ) ;
#4549=CARTESIAN_POINT ( 'NONE',  ( 24.99999999999998224, -1000.000000000000000, -138.9999999999999716 ) ) ;
#4553=FACE_BOUND ( 'NONE', #10381, .T. ) ;
#4561=ADVANCED_FACE ( 'NONE', ( #2869, #21359 ), #10047, .T. ) ;
#4565=EDGE_LOOP ( 'NONE', ( #9116, #9718 ) ) ;
#4614=ORIENTED_EDGE ( 'NONE', *, *, #7106, .T. ) ;
#4626=FILL_AREA_STYLE_COLOUR ( '', #8104 ) ;
#4627=MECHANICAL_DESIGN_GEOMETRIC_PRESENTATION_REPRESENTATION('',(#1161),#13538);
#4629=CIRCLE ( 'NONE', #14678, 20.00000000000000000 ) ;
#4638=EDGE_CURVE ( 'NONE', #13229, #14636, #20254, .T. ) ;
#4644=CARTESIAN_POINT ( 'NONE',  ( 25.00000000000000000, -1.196402736354634486E-15, -145.0000119999999697 ) ) ;
#4647=LINE ( 'NONE', #4876, #1521 ) ;
#4656=CARTESIAN_POINT ( 'NONE',  ( 1.642023387316846605, 25.00004926070564082, -145.0000000000000000 ) ) ;
#4658=( NAMED_UNIT ( * ) SI_UNIT ( $, .STERADIAN. ) SOLID_ANGLE_UNIT ( ) );
#4672=CARTESIAN_POINT ( 'NONE',  ( 0.000000000000000000, 0.000000000000000000, 124.9999999999999716 ) ) ;
#4675=CARTESIAN_POINT ( 'NONE',  ( 100.0000000000000000, 0.000000000000000000, 0.000000000000000000 ) ) ;
#4677=DIRECTION ( 'NONE',  ( 0.000000000000000000, 1.177509268541832635E-16, -1.000000000000000000 ) ) ;
#4682=ORIENTED_EDGE ( 'NONE', *, *, #12724, .T. ) ;
#4686=CARTESIAN_POINT ( 'NONE',  ( -22.46856765566313996, -1011.084098757902211, -145.0000000000001421 ) ) ;
#4691=VERTEX_POINT ( 'NONE', #18634 ) ;
#4692=DIRECTION ( 'NONE',  ( 0.000000000000000000, 1.000000000000000000, 0.000000000000000000 ) ) ;
#4728=EDGE_CURVE ( 'NONE', #3347, #21577, #13357, .T. ) ;
#4762=CARTESIAN_POINT ( 'NONE',  ( 23.72540896990116721, 8.050072860352383231, -145.0000000000000000 ) ) ;
#4785=DIRECTION ( 'NONE',  ( 0.000000000000000000, 1.000000000000000000, 0.000000000000000000 ) ) ;
#4791=CARTESIAN_POINT ( 'NONE',  ( 100.0000000000000000, -1400.000000000000000, -125.0000000000001705 ) ) ;
#4803=AXIS2_PLACEMENT_3D ( 'NONE', #3179, #23705, #19729 ) ;
#4824=EDGE_CURVE ( 'NONE', #3770, #13850, #4854, .T. ) ;
#4838=CARTESIAN_POINT ( 'NONE',  ( -24.99999999999999645, 9.326071307568738836E-16, -145.0000059999999849 ) ) ;
#4841=FACE_BOUND ( 'NONE', #5806, .T. ) ;
#4854=CIRCLE ( 'NONE', #5630, 20.00000000000000000 ) ;
#4858=CARTESIAN_POINT ( 'NONE',  ( 45.00000000000000000, 250.0000000000000000, -5.249999999999956479 ) ) ;
#4876=CARTESIAN_POINT ( 'NONE',  ( 100.0000000000000000, -1400.000000000000000, 124.9999999999998295 ) ) ;
#4893=EDGE_CURVE ( 'NONE', #22939, #13850, #6224, .T. ) ;
#4896=CIRCLE ( 'NONE', #2183, 5.249999999999973355 ) ;
#4904=EDGE_CURVE ( 'NONE', #11935, #12660, #18042, .T. ) ;
#4925=ORIENTED_EDGE ( 'NONE', *, *, #5488, .F. ) ;
#4961=VERTEX_POINT ( 'NONE', #8753 ) ;
#4994=CARTESIAN_POINT ( 'NONE',  ( 45.00000000000000000, 250.0000000000000000, 5.249999999999956479 ) ) ;
#5036=CIRCLE ( 'NONE', #7736, 5.249999999999949374 ) ;
#5064=DIRECTION ( 'NONE',  ( 0.000000000000000000, 1.177509268541832635E-16, -1.000000000000000000 ) ) ;
#5078=EDGE_CURVE ( 'NONE', #13410, #12660, #8384, .T. ) ;
#5084=DIRECTION ( 'NONE',  ( 0.000000000000000000, -1.000000000000000000, -1.177509268541832635E-16 ) ) ;
#5107=LINE ( 'NONE', #3278, #23525 ) ;
#5116=EDGE_CURVE ( 'NONE', #3094, #19888, #21883, .T. ) ;
#5126=CARTESIAN_POINT ( 'NONE',  ( 100.0000000000000000, -1420.000000000000000, 144.9999999999998295 ) ) ;
#5156=FACE_OUTER_BOUND ( 'NONE', #18447, .T. ) ;
#5172=CARTESIAN_POINT ( 'NONE',  ( -40.00000000000000000, 100.0000000000000000, -145.0000000000000284 ) ) ;
#5184=AXIS2_PLACEMENT_3D ( 'NONE', #4791, #691, #12204 ) ;
#5213=AXIS2_PLACEMENT_3D ( 'NONE', #18430, #9158, #10637 ) ;
#5233=ORIENTED_EDGE ( 'NONE', *, *, #18462, .F. ) ;
#5237=VERTEX_POINT ( 'NONE', #13605 ) ;
#5238=VECTOR ( 'NONE', #13632, 1000.000000000000000 ) ;
#5249=VERTEX_POINT ( 'NONE', #4496 ) ;
#5270=CARTESIAN_POINT ( 'NONE',  ( 34.75000000000005684, 100.0000000000000000, -145.0000000000000284 ) ) ;
#5277=ORIENTED_EDGE ( 'NONE', *, *, #11315, .F. ) ;
#5285=CARTESIAN_POINT ( 'NONE',  ( 0.000000000000000000, -1000.000000000000000, -145.0000119999999697 ) ) ;
#5306=CARTESIAN_POINT ( 'NONE',  ( 8.055391459054622061, -23.72315261474502890, 145.0000119999999697 ) ) ;
#5309=AXIS2_PLACEMENT_3D ( 'NONE', #3111, #17848, #4692 ) ;
#5319=ADVANCED_FACE ( 'NONE', ( #20546, #11415 ), #18726, .F. ) ;
#5326=CARTESIAN_POINT ( 'NONE',  ( -6.482064212728073649, -1024.200416217147222, 145.0000119999999697 ) ) ;
#5327=CYLINDRICAL_SURFACE ( 'NONE', #4164, 25.00000000000000000 ) ;
#5329=VECTOR ( 'NONE', #11835, 1000.000000000000000 ) ;
#5381=CARTESIAN_POINT ( 'NONE',  ( -72.64999999999996305, -87.33333333333338544, 148.0000000000000000 ) ) ;
#5400=CARTESIAN_POINT ( 'NONE',  ( -19.87769063953887283, 15.24974479720506437, 145.0000119999999981 ) ) ;
#5405=DIRECTION ( 'NONE',  ( 0.000000000000000000, 1.000000000000000000, 0.000000000000000000 ) ) ;
#5442=VERTEX_POINT ( 'NONE', #10437 ) ;
#5445=DIRECTION ( 'NONE',  ( 1.000000000000000000, 0.000000000000000000, 0.000000000000000000 ) ) ;
#5449=CARTESIAN_POINT ( 'NONE',  ( -22.47082401081929959, -1011.078780159199823, 145.0000119999999981 ) ) ;
#5464=ADVANCED_FACE ( 'NONE', ( #21505 ), #1339, .F. ) ;
#5465=DIRECTION ( 'NONE',  ( 0.000000000000000000, 1.177509268541832635E-16, -1.000000000000000000 ) ) ;
#5466=CYLINDRICAL_SURFACE ( 'NONE', #14579, 20.00000000000000000 ) ;
#5476=CARTESIAN_POINT ( 'NONE',  ( 16.51654882469417629, -981.1612794305008265, -145.0000000000001421 ) ) ;
#5479=CARTESIAN_POINT ( 'NONE',  ( -100.0000000000000000, -1400.000000000000000, 124.9999999999998295 ) ) ;
#5488=EDGE_CURVE ( 'NONE', #1314, #10702, #3730, .T. ) ;
#5493=EDGE_CURVE ( 'NONE', #7859, #13380, #7311, .T. ) ;
#5496=CARTESIAN_POINT ( 'NONE',  ( -18.83467029480909360, -983.4793312354817090, 145.0000119999999697 ) ) ;
#5497=ORIENTED_EDGE ( 'NONE', *, *, #4181, .T. ) ;
#5504=CARTESIAN_POINT ( 'NONE',  ( 24.99999999999998224, -1000.000000000000000, -145.0000060000000417 ) ) ;
#5507=CARTESIAN_POINT ( 'NONE',  ( 22.47082401081929248, 11.07878015919987824, 145.0000119999999697 ) ) ;
#5512=CARTESIAN_POINT ( 'NONE',  ( -24.99999999999999645, 9.326071307568738836E-16, -145.0000059999999849 ) ) ;
#5542=CARTESIAN_POINT ( 'NONE',  ( -18.83467029480909005, -16.52066876451828037, 145.0000119999999697 ) ) ;
#5552=ORIENTED_EDGE ( 'NONE', *, *, #12743, .T. ) ;
#5561=CARTESIAN_POINT ( 'NONE',  ( -100.0000000000000000, -1400.000000000000000, -125.0000000000001705 ) ) ;
#5580=DIRECTION ( 'NONE',  ( 0.000000000000000000, -1.000000000000000000, -1.110223024625156540E-16 ) ) ;
#5596=CARTESIAN_POINT ( 'NONE',  ( -67.34999999999996589, -112.6666666666667140, 144.9999999999999716 ) ) ;
#5610=CARTESIAN_POINT ( 'NONE',  ( -67.34999999999996589, -87.33333333333338544, 124.9999999999999858 ) ) ;
#5630=AXIS2_PLACEMENT_3D ( 'NONE', #22862, #6093, #4401 ) ;
#5632=ORIENTED_EDGE ( 'NONE', *, *, #22787, .T. ) ;
#5653=PRODUCT_CONTEXT ( 'NONE', #20475, 'mechanical' ) ;
#5660=ORIENTED_EDGE ( 'NONE', *, *, #14325, .T. ) ;
#5662=CARTESIAN_POINT ( 'NONE',  ( -6.482064212728082531, -24.20041621714725011, 145.0000119999999697 ) ) ;
#5683=ORIENTED_EDGE ( 'NONE', *, *, #10708, .T. ) ;
#5685=AXIS2_PLACEMENT_3D ( 'NONE', #8743, #21055, #4512 ) ;
#5710=ADVANCED_FACE ( 'NONE', ( #13444 ), #247, .F. ) ;
#5716=ADVANCED_FACE ( 'NONE', ( #17154, #16909 ), #6168, .T. ) ;
#5718=VECTOR ( 'NONE', #2043, 1000.000000000000000 ) ;
#5726=FACE_OUTER_BOUND ( 'NONE', #9930, .T. ) ;
#5727=EDGE_CURVE ( 'NONE', #20258, #19773, #4629, .T. ) ;
#5730=DIRECTION ( 'NONE',  ( -0.000000000000000000, -0.000000000000000000, 1.000000000000000000 ) ) ;
#5733=ORIENTED_EDGE ( 'NONE', *, *, #2270, .F. ) ;
#5734=CARTESIAN_POINT ( 'NONE',  ( 3.272451888078286686, -975.1611521969856540, 145.0000119999999981 ) ) ;
#5763=CARTESIAN_POINT ( 'NONE',  ( 100.0000000000000000, -1420.000000000000000, -145.0000000000001705 ) ) ;
#5779=DIRECTION ( 'NONE',  ( 1.000000000000000000, 0.000000000000000000, 0.000000000000000000 ) ) ;
#5788=AXIS2_PLACEMENT_3D ( 'NONE', #2718, #8270, #1003 ) ;
#5806=EDGE_LOOP ( 'NONE', ( #20737, #15392 ) ) ;
#5810=DIRECTION ( 'NONE',  ( 0.000000000000000000, 1.177509268541832635E-16, -1.000000000000000000 ) ) ;
#5814=CARTESIAN_POINT ( 'NONE',  ( -12.52876685377501786, -1021.695789975588468, 145.0000119999999981 ) ) ;
#5823=ORIENTED_EDGE ( 'NONE', *, *, #10769, .T. ) ;
#5846=DIRECTION ( 'NONE',  ( -0.000000000000000000, -0.000000000000000000, 1.000000000000000000 ) ) ;
#5853=ORIENTED_EDGE ( 'NONE', *, *, #1825, .T. ) ;
#5907=DIRECTION ( 'NONE',  ( -1.000000000000000000, -0.000000000000000000, -0.000000000000000000 ) ) ;
#5908=LINE ( 'NONE', #4085, #12534 ) ;
#5912=AXIS2_PLACEMENT_3D ( 'NONE', #7907, #15293, #13510 ) ;
#5938=ORIENTED_EDGE ( 'NONE', *, *, #9057, .F. ) ;
#5944=DIRECTION ( 'NONE',  ( 0.000000000000000000, 0.000000000000000000, -1.000000000000000000 ) ) ;
#5946=CARTESIAN_POINT ( 'NONE',  ( -12.52399064350059277, -978.3009594173067853, -145.0000000000001137 ) ) ;
#5972=ORIENTED_EDGE ( 'NONE', *, *, #15084, .F. ) ;
#5990=FACE_BOUND ( 'NONE', #8015, .T. ) ;
#6007=UNCERTAINTY_MEASURE_WITH_UNIT (LENGTH_MEASURE( 1.000000000000000082E-05 ), #12146, 'distance_accuracy_value', 'NONE');
#6008=EDGE_LOOP ( 'NONE', ( #18302, #1200, #529, #10134 ) ) ;
#6022=ORIENTED_EDGE ( 'NONE', *, *, #15684, .F. ) ;
#6023=CARTESIAN_POINT ( 'NONE',  ( 100.0000000000000000, 269.9999999999999432, 125.0000000000000284 ) ) ;
#6032=ORIENTED_EDGE ( 'NONE', *, *, #13492, .F. ) ;
#6036=CARTESIAN_POINT ( 'NONE',  ( 34.75000000000005684, 100.0000000000000000, 125.0000000000000000 ) ) ;
#6037=DIRECTION ( 'NONE',  ( -0.000000000000000000, -0.000000000000000000, 1.000000000000000000 ) ) ;
#6065=CARTESIAN_POINT ( 'NONE',  ( -6.487720809262722987, -975.8007591756590955, -145.0000000000001421 ) ) ;
#6093=DIRECTION ( 'NONE',  ( 0.000000000000000000, 0.000000000000000000, 1.000000000000000000 ) ) ;
#6096=ORIENTED_EDGE ( 'NONE', *, *, #17236, .F. ) ;
#6142=EDGE_LOOP ( 'NONE', ( #15647, #10259 ) ) ;
#6144=CARTESIAN_POINT ( 'NONE',  ( 22.47082401081931735, -11.07878015919984804, 145.0000119999999697 ) ) ;
#6168=PLANE ( 'NONE',  #16977 ) ;
#6170=FACE_OUTER_BOUND ( 'NONE', #22529, .T. ) ;
#6176=EDGE_LOOP ( 'NONE', ( #3477, #19113 ) ) ;
#6197=CARTESIAN_POINT ( 'NONE',  ( 8.050035157498395932, -976.2746820519779476, -145.0000000000001421 ) ) ;
#6202=EDGE_CURVE ( 'NONE', #13850, #3770, #22758, .T. ) ;
#6205=ORIENTED_EDGE ( 'NONE', *, *, #14981, .F. ) ;
#6214=EDGE_LOOP ( 'NONE', ( #18718, #3810 ) ) ;
#6220=ORIENTED_EDGE ( 'NONE', *, *, #21929, .T. ) ;
#6224=LINE ( 'NONE', #20694, #5238 ) ;
#6226=CARTESIAN_POINT ( 'NONE',  ( 8.050035159177506117, 23.72531794756937984, -145.0000000000000000 ) ) ;
#6231=CARTESIAN_POINT ( 'NONE',  ( 20.00000000000000000, -1000.000000000000000, -150.0000000000000000 ) ) ;
#6277=CIRCLE ( 'NONE', #14785, 5.249999999999949374 ) ;
#6284=CARTESIAN_POINT ( 'NONE',  ( 0.000000000000000000, 1.865214261513747767E-15, -138.9999999999999716 ) ) ;
#6288=CARTESIAN_POINT ( 'NONE',  ( -45.00000000000000000, 269.9999999999999432, 0.000000000000000000 ) ) ;
#6292=ORIENTED_EDGE ( 'NONE', *, *, #2002, .T. ) ;
#6294=CARTESIAN_POINT ( 'NONE',  ( -18.83879023463320124, -16.51661848982829284, -145.0000000000000000 ) ) ;
#6316=CARTESIAN_POINT ( 'NONE',  ( -34.75000000000005684, 100.0000000000000000, 150.2000000000009550 ) ) ;
#6324=DIRECTION ( 'NONE',  ( -0.000000000000000000, -0.000000000000000000, 1.000000000000000000 ) ) ;
#6326=EDGE_CURVE ( 'NONE', #14669, #17715, #7079, .T. ) ;
#6331=EDGE_LOOP ( 'NONE', ( #16612, #175, #18420, #11661 ) ) ;
#6336=CARTESIAN_POINT ( 'NONE',  ( 22.46856765566318614, 11.08409875790209753, -145.0000000000000000 ) ) ;
#6343=DIRECTION ( 'NONE',  ( 1.000000000000000000, 0.000000000000000000, 0.000000000000000000 ) ) ;
#6348=DIRECTION ( 'NONE',  ( 0.000000000000000000, 0.000000000000000000, -1.000000000000000000 ) ) ;
#6349=ORIENTED_EDGE ( 'NONE', *, *, #16677, .T. ) ;
#6384=ORIENTED_EDGE ( 'NONE', *, *, #21629, .F. ) ;
#6388=DIRECTION ( 'NONE',  ( -0.000000000000000000, -0.000000000000000000, 1.000000000000000000 ) ) ;
#6390=AXIS2_PLACEMENT_3D ( 'NONE', #19528, #12109, #11994 ) ;
#6392=DIRECTION ( 'NONE',  ( 0.000000000000000000, 0.000000000000000000, -1.000000000000000000 ) ) ;
#6401=CIRCLE ( 'NONE', #2532, 5.249999999999949374 ) ;
#6446=ORIENTED_EDGE ( 'NONE', *, *, #2101, .F. ) ;
#6464=VECTOR ( 'NONE', #2574, 1000.000000000000000 ) ;
#6474=CARTESIAN_POINT ( 'NONE',  ( 100.0000000000000000, -1420.000000000000000, -145.0000000000001705 ) ) ;
#6482=EDGE_LOOP ( 'NONE', ( #16799, #8301, #17710, #7417 ) ) ;
#6489=ORIENTED_EDGE ( 'NONE', *, *, #15338, .T. ) ;
#6494=ORIENTED_EDGE ( 'NONE', *, *, #12476, .F. ) ;
#6504=VERTEX_POINT ( 'NONE', #13271 ) ;
#6506=EDGE_CURVE ( 'NONE', #218, #2340, #3040, .T. ) ;
#6528=B_SPLINE_CURVE_WITH_KNOTS ( 'NONE', 3,
 ( #4838, #15498, #22827, #22938, #965, #21140, #2886, #22711, #6294, #23059, #3011, #23191, #13595, #4362, #21024, #13951, #11769, #10289, #21269, #4484, #19321, #2669, #1088, #17413, #853, #10168, #19429, #15610, #17630, #2783, #10544, #17880, #23558, #12497 ),
 .UNSPECIFIED., .F., .F.,
 ( 4, 2, 2, 2, 2, 2, 2, 2, 2, 2, 2, 2, 2, 2, 2, 2, 4 ),
 ( 0.7500000000000000000, 0.7812500000000000000, 0.8125000000000000000, 0.8437500000000000000, 0.8750000000000000000, 0.9062500000000000000, 0.9375000000000000000, 0.9687500000000000000, 1.000000000000000000, 1.031250000000000000, 1.062500000000000000, 1.093750000000000000, 1.125000000000000000, 1.156250000000000000, 1.187500000000000000, 1.218750000000000000, 1.250000000000000000 ),
 .UNSPECIFIED. ) ;
#6571=ORIENTED_EDGE ( 'NONE', *, *, #21259, .F. ) ;
#6587=DIRECTION ( 'NONE',  ( 0.000000000000000000, 1.177509268541832635E-16, -1.000000000000000000 ) ) ;
#6599=VERTEX_POINT ( 'NONE', #19564 ) ;
#6617=DIRECTION ( 'NONE',  ( 0.000000000000000000, 0.000000000000000000, 1.000000000000000000 ) ) ;
#6618=CARTESIAN_POINT ( 'NONE',  ( 3.266795293193171634, -1024.840023195373988, -145.0000000000001137 ) ) ;
#6632=EDGE_LOOP ( 'NONE', ( #10079, #7008, #1628, #16428 ) ) ;
#6660=DIRECTION ( 'NONE',  ( 0.000000000000000000, -1.000000000000000000, -1.177509268541832635E-16 ) ) ;
#6672=VERTEX_POINT ( 'NONE', #18354 ) ;
#6707=ORIENTED_EDGE ( 'NONE', *, *, #20259, .T. ) ;
#6715=CYLINDRICAL_SURFACE ( 'NONE', #2875, 5.249999999999973355 ) ;
#6730=CARTESIAN_POINT ( 'NONE',  ( 19.87452195044109615, -1015.254575742277325, -145.0000000000001137 ) ) ;
#6731=CARTESIAN_POINT ( 'NONE',  ( 45.00000000000000000, 272.9999999999999432, 0.000000000000000000 ) ) ;
#6736=CIRCLE ( 'NONE', #23304, 20.00000000000000000 ) ;
#6751=CARTESIAN_POINT ( 'NONE',  ( 0.000000000000000000, -1000.000000000000000, -138.9999999999999716 ) ) ;
#6758=AXIS2_PLACEMENT_3D ( 'NONE', #10420, #1326, #8708 ) ;
#6790=ADVANCED_FACE ( 'NONE', ( #7380 ), #9079, .F. ) ;
#6837=CARTESIAN_POINT ( 'NONE',  ( 40.00000000000000000, 100.0000000000000000, -125.0000000000000000 ) ) ;
#6891=CIRCLE ( 'NONE', #21546, 2.649999999999999467 ) ;
#6897=AXIS2_PLACEMENT_3D ( 'NONE', #18764, #7437, #86 ) ;
#6910=ORIENTED_EDGE ( 'NONE', *, *, #14506, .F. ) ;
#6914=AXIS2_PLACEMENT_3D ( 'NONE', #6946, #19730, #21669 ) ;
#6915=DIRECTION ( 'NONE',  ( 0.000000000000000000, 0.000000000000000000, -1.000000000000000000 ) ) ;
#6919=VECTOR ( 'NONE', #6037, 1000.000000000000000 ) ;
#6941=AXIS2_PLACEMENT_3D ( 'NONE', #16559, #27, #7378 ) ;
#6946=CARTESIAN_POINT ( 'NONE',  ( -69.99999999999997158, -112.6666666666667140, 144.9999999999999716 ) ) ;
#6987=EDGE_CURVE ( 'NONE', #3347, #7088, #20133, .T. ) ;
#7000=ORIENTED_EDGE ( 'NONE', *, *, #11557, .F. ) ;
#7008=ORIENTED_EDGE ( 'NONE', *, *, #8396, .T. ) ;
#7036=ORIENTED_EDGE ( 'NONE', *, *, #13421, .F. ) ;
#7038=ORIENTED_EDGE ( 'NONE', *, *, #5488, .T. ) ;
#7068=ORIENTED_EDGE ( 'NONE', *, *, #3848, .T. ) ;
#7070=AXIS2_PLACEMENT_3D ( 'NONE', #22563, #20514, #7848 ) ;
#7073=DIRECTION ( 'NONE',  ( 0.000000000000000000, 0.000000000000000000, -1.000000000000000000 ) ) ;
#7079=LINE ( 'NONE', #19757, #19623 ) ;
#7088=VERTEX_POINT ( 'NONE', #20863 ) ;
#7105=ADVANCED_FACE ( 'NONE', ( #17118 ), #17473, .F. ) ;
#7106=EDGE_CURVE ( 'NONE', #4691, #16783, #1624, .T. ) ;
#7116=DIRECTION ( 'NONE',  ( 0.000000000000000000, 1.000000000000000000, 0.000000000000000000 ) ) ;
#7122=VERTEX_POINT ( 'NONE', #6474 ) ;
#7129=LINE ( 'NONE', #12738, #17166 ) ;
#7151=DIRECTION ( 'NONE',  ( 0.000000000000000000, 0.000000000000000000, 1.000000000000000000 ) ) ;
#7186=B_SPLINE_CURVE_WITH_KNOTS ( 'NONE', 3,
 ( #12686, #8796, #20228, #16157, #18082, #5507, #9272, #11092, #23517, #8926, #14470, #19997, #16633, #16385, #1535, #14372, #7324, #18300, #14710, #16499, #10980, #14826, #3461, #7193, #14581, #21923, #5400, #12817, #3564, #11335, #22773, #15432, #11704, #11583 ),
 .UNSPECIFIED., .F., .F.,
 ( 4, 2, 2, 2, 2, 2, 2, 2, 2, 2, 2, 2, 2, 2, 2, 2, 4 ),
 ( 0.000000000000000000, 0.03125000000000000694, 0.06250000000000000000, 0.09374999999999998612, 0.1249999999999999861, 0.1562499999999999722, 0.1874999999999999722, 0.2187500000000000000, 0.2500000000000000000, 0.2812500000000000000, 0.3125000000000000000, 0.3437500000000000000, 0.3750000000000000000, 0.4062500000000000555, 0.4375000000000000555, 0.4687500000000000555, 0.5000000000000000000 ),
 .UNSPECIFIED. ) ;
#7193=CARTESIAN_POINT ( 'NONE',  ( -15.24974479720507503, 19.87769063953886572, 145.0000119999999413 ) ) ;
#7196=CARTESIAN_POINT ( 'NONE',  ( 70.00000000000000000, -112.6666666666666714, 124.9999999999999858 ) ) ;
#7236=EDGE_LOOP ( 'NONE', ( #21374, #41, #257, #15886 ) ) ;
#7237=DIRECTION ( 'NONE',  ( -0.000000000000000000, -0.000000000000000000, 1.000000000000000000 ) ) ;
#7245=CARTESIAN_POINT ( 'NONE',  ( 24.99999999999998224, -1000.000000000000000, 145.0000059999999280 ) ) ;
#7266=CARTESIAN_POINT ( 'NONE',  ( 0.000000000000000000, 1.865214261513747767E-15, 138.9999999999999716 ) ) ;
#7278=CARTESIAN_POINT ( 'NONE',  ( 19.87444003270859483, -984.7454789927647880, -145.0000000000001421 ) ) ;
#7311=CIRCLE ( 'NONE', #6941, 2.649999999999985700 ) ;
#7324=CARTESIAN_POINT ( 'NONE',  ( 1.636246173744676291, 24.99999999999999645, 145.0000119999999697 ) ) ;
#7335=EDGE_CURVE ( 'NONE', #19715, #1314, #6277, .T. ) ;
#7338=DIRECTION ( 'NONE',  ( 1.000000000000000000, 0.000000000000000000, 0.000000000000000000 ) ) ;
#7378=DIRECTION ( 'NONE',  ( 0.000000000000000000, 1.000000000000000000, 0.000000000000000000 ) ) ;
#7380=FACE_OUTER_BOUND ( 'NONE', #11625, .T. ) ;
#7411=CARTESIAN_POINT ( 'NONE',  ( 40.00000000000000000, 100.0000000000000000, 145.0000000000000000 ) ) ;
#7417=ORIENTED_EDGE ( 'NONE', *, *, #3802, .F. ) ;
#7425=CARTESIAN_POINT ( 'NONE',  ( 11.07878015919986048, -977.5291759891807715, 145.0000119999999697 ) ) ;
#7426=EDGE_LOOP ( 'NONE', ( #12854, #11638 ) ) ;
#7429=EDGE_CURVE ( 'NONE', #13361, #4420, #18333, .T. ) ;
#7432=ORIENTED_EDGE ( 'NONE', *, *, #15684, .T. ) ;
#7436=FACE_BOUND ( 'NONE', #7426, .T. ) ;
#7437=DIRECTION ( 'NONE',  ( -0.000000000000000000, -0.000000000000000000, 1.000000000000000000 ) ) ;
#7464=VERTEX_POINT ( 'NONE', #20610 ) ;
#7478=DIRECTION ( 'NONE',  ( 0.000000000000000000, 0.000000000000000000, 1.000000000000000000 ) ) ;
#7483=CARTESIAN_POINT ( 'NONE',  ( -45.24999999999994316, 100.0000000000000000, 150.2000000000009550 ) ) ;
#7484=CARTESIAN_POINT ( 'NONE',  ( 1.636246173744687837, -1024.999999999999773, 145.0000119999999697 ) ) ;
#7514=CARTESIAN_POINT ( 'NONE',  ( 23.72540896970402358, -991.9499271393301569, -145.0000000000001421 ) ) ;
#7530=CARTESIAN_POINT ( 'NONE',  ( -20.00000000000000000, -1000.000000000000000, -138.9999999999999716 ) ) ;
#7553=FACE_OUTER_BOUND ( 'NONE', #6008, .T. ) ;
#7586=CARTESIAN_POINT ( 'NONE',  ( -24.99999999999999645, -2.129009867111508370E-15, 145.0000059999999849 ) ) ;
#7593=CARTESIAN_POINT ( 'NONE',  ( 25.00000000000000000, 4.926831259382130415E-15, 145.0000119999999697 ) ) ;
#7604=CARTESIAN_POINT ( 'NONE',  ( 11.07878015919984982, -1022.470824010819570, 145.0000119999999697 ) ) ;
#7614=CIRCLE ( 'NONE', #15736, 20.00000000000000000 ) ;
#7619=CARTESIAN_POINT ( 'NONE',  ( 0.000000000000000000, 0.000000000000000000, -125.0000000000000000 ) ) ;
#7638=CARTESIAN_POINT ( 'NONE',  ( 0.000000000000000000, -1000.000000000000000, -125.0000000000001137 ) ) ;
#7659=CARTESIAN_POINT ( 'NONE',  ( 8.055391459054620285, -976.2768473852548823, 145.0000119999999981 ) ) ;
#7663=CARTESIAN_POINT ( 'NONE',  ( -100.0000000000000000, 249.9999999999999716, 125.0000000000000284 ) ) ;
#7683=CARTESIAN_POINT ( 'NONE',  ( -45.00000000000000000, 250.0000000000000000, 0.000000000000000000 ) ) ;
#7718=CARTESIAN_POINT ( 'NONE',  ( -20.00000000000000000, 2.449293598294706513E-15, 124.9999999999999716 ) ) ;
#7736=AXIS2_PLACEMENT_3D ( 'NONE', #17820, #2832, #23238 ) ;
#7744=CARTESIAN_POINT ( 'NONE',  ( -8.050035159177529209, -1023.725317947569579, -145.0000000000001421 ) ) ;
#7767=ORIENTED_EDGE ( 'NONE', *, *, #17835, .F. ) ;
#7768=CARTESIAN_POINT ( 'NONE',  ( -100.0000000000000000, 0.000000000000000000, 0.000000000000000000 ) ) ;
#7770=CARTESIAN_POINT ( 'NONE',  ( 22.46856765586026583, -988.9159012424156572, -145.0000000000001421 ) ) ;
#7773=VERTEX_POINT ( 'NONE', #13040 ) ;
#7775=EDGE_LOOP ( 'NONE', ( #13596, #19613 ) ) ;
#7784=DIRECTION ( 'NONE',  ( 0.000000000000000000, -1.177509268541832635E-16, 1.000000000000000000 ) ) ;
#7800=EDGE_CURVE ( 'NONE', #1487, #17506, #7186, .T. ) ;
#7801=FACE_OUTER_BOUND ( 'NONE', #1173, .T. ) ;
#7807=DIRECTION ( 'NONE',  ( 1.000000000000000000, 0.000000000000000000, 0.000000000000000000 ) ) ;
#7848=DIRECTION ( 'NONE',  ( 0.000000000000000000, 1.000000000000000000, 0.000000000000000000 ) ) ;
#7850=ORIENTED_EDGE ( 'NONE', *, *, #10885, .F. ) ;
#7859=VERTEX_POINT ( 'NONE', #20583 ) ;
#7877=DIRECTION ( 'NONE',  ( -1.000000000000000000, -0.000000000000000000, -0.000000000000000000 ) ) ;
#7885=DIRECTION ( 'NONE',  ( 0.000000000000000000, -1.000000000000000000, -1.110223024625156540E-16 ) ) ;
#7906=AXIS2_PLACEMENT_3D ( 'NONE', #14632, #9318, #5445 ) ;
#7907=CARTESIAN_POINT ( 'NONE',  ( 0.000000000000000000, -1000.000000000000000, -150.0000000000000000 ) ) ;
#7912=CARTESIAN_POINT ( 'NONE',  ( -11.08409875828679247, 22.46856765550231216, -145.0000000000000000 ) ) ;
#7923=CARTESIAN_POINT ( 'NONE',  ( -20.00000000000000000, -1000.000000000000000, -150.0000000000000000 ) ) ;
#7976=DIRECTION ( 'NONE',  ( -0.000000000000000000, 1.000000000000000000, -0.000000000000000000 ) ) ;
#7977=CARTESIAN_POINT ( 'NONE',  ( 16.52066876451827682, -981.1653297051909703, 145.0000119999999981 ) ) ;
#8005=CIRCLE ( 'NONE', #21492, 5.249999999999973355 ) ;
#8006=CARTESIAN_POINT ( 'NONE',  ( -18.83872056943800288, -983.4834511752143271, -145.0000000000001421 ) ) ;
#8015=EDGE_LOOP ( 'NONE', ( #12604, #1912 ) ) ;
#8037=CARTESIAN_POINT ( 'NONE',  ( 24.19924082433664125, 6.487720809269068134, -144.9999999999999716 ) ) ;
#8054=DIRECTION ( 'NONE',  ( 0.000000000000000000, 1.177509268541832635E-16, -1.000000000000000000 ) ) ;
#8074=CARTESIAN_POINT ( 'NONE',  ( 100.0000000000000000, -1400.000000000000000, -125.0000000000001705 ) ) ;
#8087=FACE_OUTER_BOUND ( 'NONE', #10874, .T. ) ;
#8097=DIRECTION ( 'NONE',  ( 0.000000000000000000, 0.000000000000000000, -1.000000000000000000 ) ) ;
#8104=COLOUR_RGB ( '',0.8941176470588234615, 0.8941176470588234615, 0.8941176470588234615 ) ;
#8110=VECTOR ( 'NONE', #8963, 1000.000000000000000 ) ;
#8111=CIRCLE ( 'NONE', #14299, 2.649999999999999467 ) ;
#8150=EDGE_CURVE ( 'NONE', #3718, #22067, #21844, .T. ) ;
#8156=FACE_OUTER_BOUND ( 'NONE', #8430, .T. ) ;
#8169=CARTESIAN_POINT ( 'NONE',  ( -24.83992656990903569, 3.266860234290754672, -145.0000000000000000 ) ) ;
#8198=ORIENTED_EDGE ( 'NONE', *, *, #11315, .T. ) ;
#8204=ORIENTED_EDGE ( 'NONE', *, *, #18577, .T. ) ;
#8207=CARTESIAN_POINT ( 'NONE',  ( -25.00000000000000000, 1.865214261513747767E-15, 138.9999999999999716 ) ) ;
#8213=CARTESIAN_POINT ( 'NONE',  ( 24.99999999999999645, 2.463415629691065208E-15, 145.0000059999999849 ) ) ;
#8228=EDGE_LOOP ( 'NONE', ( #22078, #21384 ) ) ;
#8234=FACE_BOUND ( 'NONE', #12232, .T. ) ;
#8239=LINE ( 'NONE', #17780, #11789 ) ;
#8244=CARTESIAN_POINT ( 'NONE',  ( -25.00004926070572964, -998.3579766119668193, -145.0000000000001137 ) ) ;
#8245=EDGE_CURVE ( 'NONE', #6599, #12056, #4896, .T. ) ;
#8258=LINE ( 'NONE', #22849, #10813 ) ;
#8262=FACE_BOUND ( 'NONE', #18677, .T. ) ;
#8265=ORIENTED_EDGE ( 'NONE', *, *, #12978, .T. ) ;
#8270=DIRECTION ( 'NONE',  ( 0.000000000000000000, 1.177509268541832635E-16, -1.000000000000000000 ) ) ;
#8274=CARTESIAN_POINT ( 'NONE',  ( -23.72528575881786850, 8.050112875934637202, -145.0000000000000000 ) ) ;
#8299=DIRECTION ( 'NONE',  ( 0.000000000000000000, 1.000000000000000000, 0.000000000000000000 ) ) ;
#8301=ORIENTED_EDGE ( 'NONE', *, *, #21900, .F. ) ;
#8307=CIRCLE ( 'NONE', #5213, 5.249999999999956479 ) ;
#8311=ORIENTED_EDGE ( 'NONE', *, *, #1825, .F. ) ;
#8327=DIRECTION ( 'NONE',  ( -0.000000000000000000, -0.000000000000000000, 1.000000000000000000 ) ) ;
#8328=VERTEX_POINT ( 'NONE', #2538 ) ;
#8354=CARTESIAN_POINT ( 'NONE',  ( -24.99999999999998224, -1000.000000000000000, -145.0000060000000417 ) ) ;
#8355=VECTOR ( 'NONE', #5084, 1000.000000000000000 ) ;
#8363=PRESENTATION_STYLE_ASSIGNMENT (( #981 ) ) ;
#8376=FACE_OUTER_BOUND ( 'NONE', #15469, .T. ) ;
#8378=LINE ( 'NONE', #10204, #22336 ) ;
#8380=VERTEX_POINT ( 'NONE', #12241 ) ;
#8384=LINE ( 'NONE', #15761, #21433 ) ;
#8396=EDGE_CURVE ( 'NONE', #18735, #13410, #10416, .T. ) ;
#8404=DIRECTION ( 'NONE',  ( 0.000000000000000000, 0.000000000000000000, 1.000000000000000000 ) ) ;
#8410=AXIS2_PLACEMENT_3D ( 'NONE', #7196, #14585, #5405 ) ;
#8415=LINE ( 'NONE', #1279, #12725 ) ;
#8430=EDGE_LOOP ( 'NONE', ( #3144, #6910, #17616, #22142 ) ) ;
#8442=DIRECTION ( 'NONE',  ( -1.000000000000000000, 0.000000000000000000, 0.000000000000000000 ) ) ;
#8449=VECTOR ( 'NONE', #815, 1000.000000000000000 ) ;
#8465=EDGE_LOOP ( 'NONE', ( #11140, #391 ) ) ;
#8506=EDGE_LOOP ( 'NONE', ( #20531, #9827, #22800, #17026 ) ) ;
#8551=DIRECTION ( 'NONE',  ( 0.000000000000000000, -0.000000000000000000, 1.000000000000000000 ) ) ;
#8554=CARTESIAN_POINT ( 'NONE',  ( 15.25452100747948769, -1019.874440032434222, -145.0000000000001421 ) ) ;
#8572=DIRECTION ( 'NONE',  ( 0.000000000000000000, 0.000000000000000000, -1.000000000000000000 ) ) ;
#8582=EDGE_CURVE ( 'NONE', #17506, #1487, #10654, .T. ) ;
#8584=CARTESIAN_POINT ( 'NONE',  ( -100.0000000000000000, 249.9999999999999716, 125.0000000000000284 ) ) ;
#8588=VECTOR ( 'NONE', #13658, 1000.000000000000000 ) ;
#8605=FACE_OUTER_BOUND ( 'NONE', #16623, .T. ) ;
#8606=( LENGTH_UNIT ( ) NAMED_UNIT ( * ) SI_UNIT ( .MILLI., .METRE. ) );
#8658=DIRECTION ( 'NONE',  ( -0.000000000000000000, -0.000000000000000000, 1.000000000000000000 ) ) ;
#8685=EDGE_LOOP ( 'NONE', ( #17224, #14171 ) ) ;
#8687=ADVANCED_FACE ( 'NONE', ( #8087 ), #15335, .F. ) ;
#8708=DIRECTION ( 'NONE',  ( 0.000000000000000000, 1.000000000000000000, 0.000000000000000000 ) ) ;
#8711=ORIENTED_EDGE ( 'NONE', *, *, #431, .F. ) ;
#8715=ORIENTED_EDGE ( 'NONE', *, *, #8970, .T. ) ;
#8721=DIRECTION ( 'NONE',  ( 0.000000000000000000, 0.000000000000000000, -1.000000000000000000 ) ) ;
#8736=AXIS2_PLACEMENT_3D ( 'NONE', #9092, #20076, #3397 ) ;
#8742=EDGE_CURVE ( 'NONE', #15596, #14669, #14193, .T. ) ;
#8743=CARTESIAN_POINT ( 'NONE',  ( -40.00000000000000000, 100.0000000000000000, 150.2000000000009550 ) ) ;
#8753=CARTESIAN_POINT ( 'NONE',  ( -45.00000000000000000, 250.0000000000000000, 5.249999999999956479 ) ) ;
#8765=CARTESIAN_POINT ( 'NONE',  ( 40.00000000000000000, 100.0000000000000000, -145.0000000000000284 ) ) ;
#8781=CARTESIAN_POINT ( 'NONE',  ( 45.00000000000000000, 269.9999999999999432, 0.000000000000000000 ) ) ;
#8792=DIRECTION ( 'NONE',  ( 1.000000000000000000, 0.000000000000000000, 0.000000000000000000 ) ) ;
#8796=CARTESIAN_POINT ( 'NONE',  ( 25.00000000000000355, 1.636246173744694277, 145.0000119999999697 ) ) ;
#8811=DIRECTION ( 'NONE',  ( 0.000000000000000000, 0.000000000000000000, 1.000000000000000000 ) ) ;
#8869=DIRECTION ( 'NONE',  ( 0.000000000000000000, 1.000000000000000000, 0.000000000000000000 ) ) ;
#8870=ADVANCED_FACE ( 'NONE', ( #18200 ), #18417, .F. ) ;
#8872=FACE_OUTER_BOUND ( 'NONE', #23160, .T. ) ;
#8924=DIRECTION ( 'NONE',  ( 0.000000000000000000, -1.177509268541832635E-16, 1.000000000000000000 ) ) ;
#8926=CARTESIAN_POINT ( 'NONE',  ( 16.52066876451829103, 18.83467029480909360, 145.0000119999999697 ) ) ;
#8940=EDGE_LOOP ( 'NONE', ( #12135, #17491, #11708, #2332 ) ) ;
#8946=VERTEX_POINT ( 'NONE', #10876 ) ;
#8963=DIRECTION ( 'NONE',  ( -0.000000000000000000, -0.000000000000000000, 1.000000000000000000 ) ) ;
#8970=EDGE_CURVE ( 'NONE', #17386, #13236, #12298, .T. ) ;
#8976=EDGE_LOOP ( 'NONE', ( #19175, #9567 ) ) ;
#8981=CARTESIAN_POINT ( 'NONE',  ( 0.000000000000000000, -1000.000000000000000, -150.0000000000000000 ) ) ;
#8983=LINE ( 'NONE', #19839, #10024 ) ;
#8988=VECTOR ( 'NONE', #476, 1000.000000000000000 ) ;
#8995=CARTESIAN_POINT ( 'NONE',  ( -40.00000000000000000, 100.0000000000000000, -125.0000000000000000 ) ) ;
#9024=ADVANCED_FACE ( 'NONE', ( #2482, #14949, #22776, #562, #16857, #9870, #11827, #675, #5990 ), #11455, .F. ) ;
#9043=FACE_OUTER_BOUND ( 'NONE', #7236, .T. ) ;
#9049=ORIENTED_EDGE ( 'NONE', *, *, #17309, .T. ) ;
#9057=EDGE_CURVE ( 'NONE', #10540, #2069, #20710, .T. ) ;
#9061=CARTESIAN_POINT ( 'NONE',  ( -21.69578997558839362, -12.52876685377503563, 145.0000119999999697 ) ) ;
#9068=AXIS2_PLACEMENT_3D ( 'NONE', #96, #19021, #2491 ) ;
#9077=CARTESIAN_POINT ( 'NONE',  ( 21.69578997558838296, -1012.528766853774982, 145.0000119999999697 ) ) ;
#9079=CYLINDRICAL_SURFACE ( 'NONE', #3929, 2.649999999999999467 ) ;
#9092=CARTESIAN_POINT ( 'NONE',  ( -40.00000000000000000, 100.0000000000000000, -145.0000000000000284 ) ) ;
#9105=ORIENTED_EDGE ( 'NONE', *, *, #15084, .T. ) ;
#9107=CARTESIAN_POINT ( 'NONE',  ( 24.99999999999998224, -1000.000000000000000, -145.0000060000000417 ) ) ;
#9116=ORIENTED_EDGE ( 'NONE', *, *, #15108, .F. ) ;
#9158=DIRECTION ( 'NONE',  ( -0.000000000000000000, 1.000000000000000000, -0.000000000000000000 ) ) ;
#9199=CARTESIAN_POINT ( 'NONE',  ( -24.83884780301425721, -1003.272451888078649, 145.0000119999999981 ) ) ;
#9203=AXIS2_PLACEMENT_3D ( 'NONE', #14227, #8404, #23129 ) ;
#9206=CARTESIAN_POINT ( 'NONE',  ( -100.0000000000000000, 269.9999999999999432, 125.0000000000000284 ) ) ;
#9223=CYLINDRICAL_SURFACE ( 'NONE', #13831, 2.649999999999999467 ) ;
#9262=CARTESIAN_POINT ( 'NONE',  ( -1.636246173744689836, -974.9999999999997726, 145.0000119999999697 ) ) ;
#9272=CARTESIAN_POINT ( 'NONE',  ( 21.69578997558838651, 12.52876685377504096, 145.0000119999999697 ) ) ;
#9276=DIRECTION ( 'NONE',  ( -1.000000000000000000, 0.000000000000000000, 0.000000000000000000 ) ) ;
#9286=DIRECTION ( 'NONE',  ( 0.000000000000000000, -1.177509268541832635E-16, 1.000000000000000000 ) ) ;
#9309=CARTESIAN_POINT ( 'NONE',  ( -24.83884780301427853, -3.272451888078302229, 145.0000119999999981 ) ) ;
#9313=LINE ( 'NONE', #7593, #9539 ) ;
#9317=EDGE_LOOP ( 'NONE', ( #5277, #10044, #6571, #2006 ) ) ;
#9318=DIRECTION ( 'NONE',  ( 0.000000000000000000, 0.000000000000000000, 1.000000000000000000 ) ) ;
#9319=EDGE_CURVE ( 'NONE', #19773, #20769, #21784, .T. ) ;
#9325=CARTESIAN_POINT ( 'NONE',  ( 8.055391459054613179, -1023.723152614744777, 145.0000119999999697 ) ) ;
#9330=FACE_BOUND ( 'NONE', #19081, .T. ) ;
#9343=DIRECTION ( 'NONE',  ( 0.000000000000000000, 0.000000000000000000, 1.000000000000000000 ) ) ;
#9345=CARTESIAN_POINT ( 'NONE',  ( -100.0000000000000000, -1400.000000000000000, -125.0000000000001705 ) ) ;
#9349=ORIENTED_EDGE ( 'NONE', *, *, #11440, .T. ) ;
#9362=CARTESIAN_POINT ( 'NONE',  ( 34.75000000000005684, 100.0000000000000000, 150.2000000000009550 ) ) ;
#9382=FACE_BOUND ( 'NONE', #3663, .T. ) ;
#9403=DIRECTION ( 'NONE',  ( 0.000000000000000000, 0.000000000000000000, 1.000000000000000000 ) ) ;
#9426=AXIS2_PLACEMENT_3D ( 'NONE', #7411, #2192, #1967 ) ;
#9473=CARTESIAN_POINT ( 'NONE',  ( 0.000000000000000000, 0.000000000000000000, 0.000000000000000000 ) ) ;
#9476=EDGE_CURVE ( 'NONE', #20600, #15247, #15837, .T. ) ;
#9496=ORIENTED_EDGE ( 'NONE', *, *, #2472, .T. ) ;
#9509=ORIENTED_EDGE ( 'NONE', *, *, #11867, .T. ) ;
#9530=ORIENTED_EDGE ( 'NONE', *, *, #5727, .T. ) ;
#9532=DIRECTION ( 'NONE',  ( -0.000000000000000000, -0.000000000000000000, 1.000000000000000000 ) ) ;
#9539=VECTOR ( 'NONE', #11371, 1000.000000000000000 ) ;
#9540=DIRECTION ( 'NONE',  ( 0.000000000000000000, 0.000000000000000000, 1.000000000000000000 ) ) ;
#9551=CARTESIAN_POINT ( 'NONE',  ( 24.99999999999997868, -998.3637538262552198, 145.0000119999999697 ) ) ;
#9555=DIRECTION ( 'NONE',  ( -1.000000000000000000, 0.000000000000000000, 0.000000000000000000 ) ) ;
#9567=ORIENTED_EDGE ( 'NONE', *, *, #2002, .F. ) ;
#9587=CARTESIAN_POINT ( 'NONE',  ( 70.00000000000000000, -112.6666666666666714, 144.9999999999999716 ) ) ;
#9591=CIRCLE ( 'NONE', #719, 2.649999999999999467 ) ;
#9653=DIRECTION ( 'NONE',  ( 0.000000000000000000, 0.000000000000000000, 1.000000000000000000 ) ) ;
#9654=LINE ( 'NONE', #22658, #16921 ) ;
#9667=EDGE_CURVE ( 'NONE', #17506, #14601, #16577, .T. ) ;
#9673=AXIS2_PLACEMENT_3D ( 'NONE', #8781, #18068, #7073 ) ;
#9677=ORIENTED_EDGE ( 'NONE', *, *, #17560, .T. ) ;
#9682=LINE ( 'NONE', #2525, #21010 ) ;
#9705=LINE ( 'NONE', #13350, #3084 ) ;
#9718=ORIENTED_EDGE ( 'NONE', *, *, #13348, .F. ) ;
#9723=EDGE_CURVE ( 'NONE', #4961, #12056, #5107, .T. ) ;
#9743=CARTESIAN_POINT ( 'NONE',  ( 40.00000000000000000, 100.0000000000000000, -125.0000000000000000 ) ) ;
#9776=ORIENTED_EDGE ( 'NONE', *, *, #8245, .F. ) ;
#9783=DIRECTION ( 'NONE',  ( 0.000000000000000000, -1.110223024625156540E-16, 1.000000000000000000 ) ) ;
#9792=CARTESIAN_POINT ( 'NONE',  ( 70.00000000000000000, -87.33333333333332860, 145.0000000000000000 ) ) ;
#9797=DIRECTION ( 'NONE',  ( 0.000000000000000000, 0.000000000000000000, -1.000000000000000000 ) ) ;
#9799=CARTESIAN_POINT ( 'NONE',  ( -11.08413645907697820, -1022.468658677994995, -145.0000000000001137 ) ) ;
#9827=ORIENTED_EDGE ( 'NONE', *, *, #490, .F. ) ;
#9837=EDGE_LOOP ( 'NONE', ( #6096, #23109, #12406, #6205 ) ) ;
#9846=DIRECTION ( 'NONE',  ( -0.000000000000000000, -0.000000000000000000, 1.000000000000000000 ) ) ;
#9859=CARTESIAN_POINT ( 'NONE',  ( 19.87444003266270087, 15.25452100728112015, -145.0000000000000000 ) ) ;
#9867=DIRECTION ( 'NONE',  ( -0.000000000000000000, -0.000000000000000000, 1.000000000000000000 ) ) ;
#9870=FACE_BOUND ( 'NONE', #1578, .T. ) ;
#9874=AXIS2_PLACEMENT_3D ( 'NONE', #23029, #1302, #8442 ) ;
#9900=ADVANCED_FACE ( 'NONE', ( #20533 ), #18712, .F. ) ;
#9921=DIRECTION ( 'NONE',  ( -0.000000000000000000, -0.000000000000000000, 1.000000000000000000 ) ) ;
#9930=EDGE_LOOP ( 'NONE', ( #13703, #11808, #12810, #22851 ) ) ;
#9967=CARTESIAN_POINT ( 'NONE',  ( -69.99999999999997158, -87.33333333333338544, 148.0000000000000000 ) ) ;
#9969=B_SPLINE_CURVE_WITH_KNOTS ( 'NONE', 3,
 ( #9107, #16710, #16946, #20088, #7514, #7770, #20189, #7278, #22016, #5476, #12884, #3641, #17424, #6197, #22483, #17184, #11534, #975, #15511, #6065, #13832, #4497, #5946, #22837, #755, #8006, #13355, #15620, #20669, #13482, #864, #21155, #8244, #8354 ),
 .UNSPECIFIED., .F., .F.,
 ( 4, 2, 2, 2, 2, 2, 2, 2, 2, 2, 2, 2, 2, 2, 2, 2, 4 ),
 ( 0.2500000000000000000, 0.2812500000000000000, 0.3125000000000000000, 0.3437500000000000000, 0.3750000000000000000, 0.4062500000000000000, 0.4375000000000000000, 0.4687500000000000000, 0.5000000000000000000, 0.5312500000000000000, 0.5625000000000000000, 0.5937500000000000000, 0.6250000000000000000, 0.6562500000000000000, 0.6875000000000000000, 0.7187500000000000000, 0.7500000000000000000 ),
 .UNSPECIFIED. ) ;
#9970=PLANE ( 'NONE',  #18450 ) ;
#9976=CARTESIAN_POINT ( 'NONE',  ( 0.000000000000000000, -1000.000000000000000, -150.0000000000000000 ) ) ;
#10011=DIRECTION ( 'NONE',  ( 0.000000000000000000, -1.000000000000000000, 0.000000000000000000 ) ) ;
#10024=VECTOR ( 'NONE', #7151, 1000.000000000000000 ) ;
#10044=ORIENTED_EDGE ( 'NONE', *, *, #2023, .T. ) ;
#10047=PLANE ( 'NONE',  #14130 ) ;
#10061=ORIENTED_EDGE ( 'NONE', *, *, #11367, .F. ) ;
#10079=ORIENTED_EDGE ( 'NONE', *, *, #18935, .T. ) ;
#10084=DIRECTION ( 'NONE',  ( 1.000000000000000000, 0.000000000000000000, 0.000000000000000000 ) ) ;
#10119=DIRECTION ( 'NONE',  ( -1.000000000000000000, 0.000000000000000000, 0.000000000000000000 ) ) ;
#10134=ORIENTED_EDGE ( 'NONE', *, *, #15976, .T. ) ;
#10142=EDGE_LOOP ( 'NONE', ( #20301, #18301, #23337, #9776 ) ) ;
#10168=CARTESIAN_POINT ( 'NONE',  ( 18.83866108960308949, -16.51660830817425207, -145.0000000000000000 ) ) ;
#10171=DIRECTION ( 'NONE',  ( 0.000000000000000000, 1.177509268541832635E-16, -1.000000000000000000 ) ) ;
#10188=SURFACE_STYLE_FILL_AREA ( #12046 ) ;
#10194=AXIS2_PLACEMENT_3D ( 'NONE', #17719, #4092, #18820 ) ;
#10204=CARTESIAN_POINT ( 'NONE',  ( 24.99999999999998224, -1000.000000000000000, 145.0000119999999697 ) ) ;
#10211=CIRCLE ( 'NONE', #12949, 20.00000000000001776 ) ;
#10218=ADVANCED_FACE ( 'NONE', ( #567 ), #2120, .F. ) ;
#10231=DIRECTION ( 'NONE',  ( -1.000000000000000000, 0.000000000000000000, 0.000000000000000000 ) ) ;
#10232=FACE_OUTER_BOUND ( 'NONE', #12049, .T. ) ;
#10248=CARTESIAN_POINT ( 'NONE',  ( 100.0000000000000000, -1400.000000000000000, 124.9999999999998295 ) ) ;
#10253=CARTESIAN_POINT ( 'NONE',  ( -1.641270926519074580, -1025.000000000000227, -145.0000000000001137 ) ) ;
#10259=ORIENTED_EDGE ( 'NONE', *, *, #12978, .F. ) ;
#10273=ORIENTED_EDGE ( 'NONE', *, *, #3119, .F. ) ;
#10275=CARTESIAN_POINT ( 'NONE',  ( -100.0000000000000000, 249.9999999999999716, 145.0000000000000284 ) ) ;
#10289=CARTESIAN_POINT ( 'NONE',  ( 1.641270926519074136, -24.99999999999991118, -145.0000000000000000 ) ) ;
#10293=FACE_BOUND ( 'NONE', #7775, .T. ) ;
#10295=AXIS2_PLACEMENT_3D ( 'NONE', #19978, #1394, #14454 ) ;
#10317=ORIENTED_EDGE ( 'NONE', *, *, #6987, .F. ) ;
#10367=PLANE ( 'NONE',  #5184 ) ;
#10371=AXIS2_PLACEMENT_3D ( 'NONE', #19976, #20206, #18392 ) ;
#10381=EDGE_LOOP ( 'NONE', ( #19184, #6446 ) ) ;
#10394=ORIENTED_EDGE ( 'NONE', *, *, #13421, .T. ) ;
#10408=VECTOR ( 'NONE', #21861, 1000.000000000000000 ) ;
#10416=LINE ( 'NONE', #8584, #8355 ) ;
#10420=CARTESIAN_POINT ( 'NONE',  ( 70.00000000000000000, -112.6666666666666714, 144.9999999999999716 ) ) ;
#10424=ORIENTED_EDGE ( 'NONE', *, *, #22935, .F. ) ;
#10429=FACE_BOUND ( 'NONE', #15098, .T. ) ;
#10437=CARTESIAN_POINT ( 'NONE',  ( -100.0000000000000000, 250.0000000000000000, -124.9999999999999716 ) ) ;
#10450=ORIENTED_EDGE ( 'NONE', *, *, #940, .T. ) ;
#10473=( NAMED_UNIT ( * ) PLANE_ANGLE_UNIT ( ) SI_UNIT ( $, .RADIAN. ) );
#10476=CARTESIAN_POINT ( 'NONE',  ( 45.24999999999994316, 100.0000000000000000, -125.0000000000000000 ) ) ;
#10479=ADVANCED_FACE ( 'NONE', ( #23366 ), #2835, .F. ) ;
#10507=DIRECTION ( 'NONE',  ( 0.000000000000000000, 0.000000000000000000, 1.000000000000000000 ) ) ;
#10540=VERTEX_POINT ( 'NONE', #7530 ) ;
#10544=CARTESIAN_POINT ( 'NONE',  ( 24.19933745025248228, -6.487655866515820158, -145.0000000000000000 ) ) ;
#10593=DIRECTION ( 'NONE',  ( 0.000000000000000000, -1.177509268541832635E-16, 1.000000000000000000 ) ) ;
#10637=DIRECTION ( 'NONE',  ( 0.000000000000000000, 0.000000000000000000, 1.000000000000000000 ) ) ;
#10642=DIRECTION ( 'NONE',  ( -0.000000000000000000, 1.000000000000000000, -0.000000000000000000 ) ) ;
#10654=B_SPLINE_CURVE_WITH_KNOTS ( 'NONE', 3,
 ( #7586, #22075, #9309, #16660, #20148, #3494, #9061, #11015, #5542, #18335, #22189, #1788, #115, #14979, #5662, #10773, #16537, #16421, #13073, #1572, #5306, #21840, #20504, #12720, #20039, #6, #13569, #356, #6144, #4203, #20879, #18800, #4333, #19167 ),
 .UNSPECIFIED., .F., .F.,
 ( 4, 2, 2, 2, 2, 2, 2, 2, 2, 2, 2, 2, 2, 2, 2, 2, 4 ),
 ( 0.5000000000000000000, 0.5312500000000000000, 0.5625000000000000000, 0.5937500000000000000, 0.6250000000000000000, 0.6562500000000000000, 0.6875000000000000000, 0.7187500000000000000, 0.7500000000000000000, 0.7812500000000000000, 0.8125000000000000000, 0.8437500000000000000, 0.8750000000000000000, 0.9062500000000000000, 0.9375000000000000000, 0.9687500000000000000, 1.000000000000000000 ),
 .UNSPECIFIED. ) ;
#10675=AXIS2_PLACEMENT_3D ( 'NONE', #7768, #22481, #5944 ) ;
#10699=ORIENTED_EDGE ( 'NONE', *, *, #5493, .F. ) ;
#10702=VERTEX_POINT ( 'NONE', #15524 ) ;
#10708=EDGE_CURVE ( 'NONE', #17386, #8380, #8258, .T. ) ;
#10726=ORIENTED_EDGE ( 'NONE', *, *, #15767, .F. ) ;
#10769=EDGE_CURVE ( 'NONE', #21577, #2989, #11918, .T. ) ;
#10773=CARTESIAN_POINT ( 'NONE',  ( -3.272451888078292903, -24.83884780301427497, 145.0000120000000265 ) ) ;
#10786=MECHANICAL_DESIGN_GEOMETRIC_PRESENTATION_REPRESENTATION('',(#735),#22710);
#10802=ORIENTED_EDGE ( 'NONE', *, *, #8245, .T. ) ;
#10805=VECTOR ( 'NONE', #20662, 1000.000000000000000 ) ;
#10813=VECTOR ( 'NONE', #13731, 1000.000000000000000 ) ;
#10836=AXIS2_PLACEMENT_3D ( 'NONE', #13584, #22816, #13217 ) ;
#10856=CARTESIAN_POINT ( 'NONE',  ( -34.75000000000005684, 100.0000000000000000, 145.0000000000000000 ) ) ;
#10869=CARTESIAN_POINT ( 'NONE',  ( 25.00004926070572253, -1001.642023387835820, -145.0000000000001137 ) ) ;
#10874=EDGE_LOOP ( 'NONE', ( #19358, #11211, #10061, #20476 ) ) ;
#10876=CARTESIAN_POINT ( 'NONE',  ( 24.99999999999999645, -5.982013681773172432E-16, -145.0000059999999849 ) ) ;
#10885=EDGE_CURVE ( 'NONE', #2113, #14636, #15127, .T. ) ;
#10893=ORIENTED_EDGE ( 'NONE', *, *, #11367, .T. ) ;
#10914=CARTESIAN_POINT ( 'NONE',  ( 18.83467029480908650, -1016.520668764518064, 145.0000119999999697 ) ) ;
#10932=EDGE_CURVE ( 'NONE', #20062, #2118, #21965, .T. ) ;
#10939=DIRECTION ( 'NONE',  ( 0.000000000000000000, 0.000000000000000000, -1.000000000000000000 ) ) ;
#10976=CARTESIAN_POINT ( 'NONE',  ( 24.83992656992418446, -1003.266860234099909, -145.0000000000001421 ) ) ;
#10979=CARTESIAN_POINT ( 'NONE',  ( -72.64999999999996305, -87.33333333333338544, 124.9999999999999858 ) ) ;
#10980=CARTESIAN_POINT ( 'NONE',  ( -8.055391459054618508, 23.72315261474503600, 145.0000119999999697 ) ) ;
#10990=CARTESIAN_POINT ( 'NONE',  ( 0.000000000000000000, -1000.000000000000000, 138.9999999999999716 ) ) ;
#11015=CARTESIAN_POINT ( 'NONE',  ( -19.87769063953886217, -15.24974479720506970, 145.0000119999999981 ) ) ;
#11067=DIRECTION ( 'NONE',  ( 0.000000000000000000, 0.000000000000000000, 1.000000000000000000 ) ) ;
#11075=DIRECTION ( 'NONE',  ( 0.000000000000000000, 0.000000000000000000, 1.000000000000000000 ) ) ;
#11080=CARTESIAN_POINT ( 'NONE',  ( -12.52876685377503385, -978.3042100244115318, 145.0000119999999697 ) ) ;
#11092=CARTESIAN_POINT ( 'NONE',  ( 19.87769063953886217, 15.24974479720507325, 145.0000119999999981 ) ) ;
#11104=ORIENTED_EDGE ( 'NONE', *, *, #3119, .T. ) ;
#11105=FACE_OUTER_BOUND ( 'NONE', #3391, .T. ) ;
#11126=CARTESIAN_POINT ( 'NONE',  ( 40.00000000000000000, 100.0000000000000000, 150.2000000000009550 ) ) ;
#11131=AXIS2_PLACEMENT_3D ( 'NONE', #7266, #14540, #21874 ) ;
#11140=ORIENTED_EDGE ( 'NONE', *, *, #3434, .F. ) ;
#11155=CIRCLE ( 'NONE', #14986, 20.00000000000000000 ) ;
#11170=ORIENTED_EDGE ( 'NONE', *, *, #3725, .F. ) ;
#11186=DIRECTION ( 'NONE',  ( -0.000000000000000000, -0.000000000000000000, 1.000000000000000000 ) ) ;
#11189=DIRECTION ( 'NONE',  ( 0.000000000000000000, -1.000000000000000000, 0.000000000000000000 ) ) ;
#11204=ADVANCED_FACE ( 'NONE', ( #2580 ), #546, .F. ) ;
#11210=AXIS2_PLACEMENT_3D ( 'NONE', #9473, #14914, #3769 ) ;
#11211=ORIENTED_EDGE ( 'NONE', *, *, #20627, .T. ) ;
#11214=CARTESIAN_POINT ( 'NONE',  ( 6.482064212728070096, -975.7995837828526646, 145.0000119999999697 ) ) ;
#11225=CARTESIAN_POINT ( 'NONE',  ( -40.00000000000000000, 100.0000000000000000, -125.0000000000000000 ) ) ;
#11278=LINE ( 'NONE', #18587, #5718 ) ;
#11298=FACE_OUTER_BOUND ( 'NONE', #16364, .T. ) ;
#11308=CARTESIAN_POINT ( 'NONE',  ( 72.64999999999999147, -87.33333333333332860, 124.9999999999999858 ) ) ;
#11315=EDGE_CURVE ( 'NONE', #16783, #4691, #20608, .T. ) ;
#11324=CARTESIAN_POINT ( 'NONE',  ( -24.99999999999998224, -998.3637538262555609, 145.0000119999999697 ) ) ;
#11335=CARTESIAN_POINT ( 'NONE',  ( -23.72315261474503600, 8.055391459054607850, 145.0000119999999697 ) ) ;
#11346=ORIENTED_EDGE ( 'NONE', *, *, #3802, .T. ) ;
#11355=DIRECTION ( 'NONE',  ( 0.000000000000000000, 1.000000000000000000, 0.000000000000000000 ) ) ;
#11367=EDGE_CURVE ( 'NONE', #4420, #16878, #11396, .T. ) ;
#11368=ADVANCED_FACE ( 'NONE', ( #20632 ), #22332, .F. ) ;
#11371=DIRECTION ( 'NONE',  ( 0.000000000000000000, 0.000000000000000000, -1.000000000000000000 ) ) ;
#11377=CIRCLE ( 'NONE', #4803, 20.00000000000000000 ) ;
#11385=CARTESIAN_POINT ( 'NONE',  ( -23.72315261474500758, -1008.055391459054704, 145.0000119999999697 ) ) ;
#11396=CIRCLE ( 'NONE', #23696, 2.649999999999999467 ) ;
#11413=AXIS2_PLACEMENT_3D ( 'NONE', #485, #2148, #9540 ) ;
#11415=FACE_BOUND ( 'NONE', #6632, .T. ) ;
#11426=ORIENTED_EDGE ( 'NONE', *, *, #15938, .F. ) ;
#11433=DIRECTION ( 'NONE',  ( 1.000000000000000000, 0.000000000000000000, 0.000000000000000000 ) ) ;
#11436=CARTESIAN_POINT ( 'NONE',  ( -22.47082401081930314, -988.9212198408002905, 145.0000119999999697 ) ) ;
#11439=DIRECTION ( 'NONE',  ( 0.000000000000000000, 1.000000000000000000, 0.000000000000000000 ) ) ;
#11440=EDGE_CURVE ( 'NONE', #7122, #21239, #5908, .T. ) ;
#11455=PLANE ( 'NONE',  #21890 ) ;
#11493=VECTOR ( 'NONE', #13056, 1000.000000000000000 ) ;
#11534=CARTESIAN_POINT ( 'NONE',  ( 1.642023387942651569, -974.9999507392942633, -145.0000000000001137 ) ) ;
#11538=ORIENTED_EDGE ( 'NONE', *, *, #12300, .F. ) ;
#11557=EDGE_CURVE ( 'NONE', #7464, #3094, #21006, .T. ) ;
#11583=CARTESIAN_POINT ( 'NONE',  ( -24.99999999999999645, -2.129009867111508370E-15, 145.0000059999999849 ) ) ;
#11605=LINE ( 'NONE', #17241, #1500 ) ;
#11622=AXIS2_PLACEMENT_3D ( 'NONE', #13649, #4044, #20587 ) ;
#11625=EDGE_LOOP ( 'NONE', ( #8711, #3212, #16149, #7850 ) ) ;
#11628=ADVANCED_FACE ( 'NONE', ( #1068 ), #948, .F. ) ;
#11633=AXIS2_PLACEMENT_3D ( 'NONE', #3612, #1809, #18356 ) ;
#11637=VECTOR ( 'NONE', #5846, 1000.000000000000000 ) ;
#11638=ORIENTED_EDGE ( 'NONE', *, *, #12300, .T. ) ;
#11640=ORIENTED_EDGE ( 'NONE', *, *, #16063, .T. ) ;
#11641=ORIENTED_EDGE ( 'NONE', *, *, #8742, .T. ) ;
#11644=LINE ( 'NONE', #23016, #17886 ) ;
#11646=CARTESIAN_POINT ( 'NONE',  ( 22.47082401081927827, -988.9212198408001768, 145.0000119999999981 ) ) ;
#11661=ORIENTED_EDGE ( 'NONE', *, *, #19638, .F. ) ;
#11704=CARTESIAN_POINT ( 'NONE',  ( -24.99999999999999289, 1.636246173744676291, 145.0000119999999697 ) ) ;
#11708=ORIENTED_EDGE ( 'NONE', *, *, #17996, .F. ) ;
#11711=CARTESIAN_POINT ( 'NONE',  ( 0.000000000000000000, 0.000000000000000000, -150.0000000000000000 ) ) ;
#11758=CARTESIAN_POINT ( 'NONE',  ( -40.00000000000000000, 100.0000000000000000, 150.2000000000009550 ) ) ;
#11759=CARTESIAN_POINT ( 'NONE',  ( 15.24974479720504661, -980.1223093604610312, 145.0000119999999697 ) ) ;
#11769=CARTESIAN_POINT ( 'NONE',  ( -1.641270926519074580, -24.99999999999990763, -145.0000000000000000 ) ) ;
#11789=VECTOR ( 'NONE', #6660, 1000.000000000000000 ) ;
#11792=VECTOR ( 'NONE', #11075, 1000.000000000000000 ) ;
#11808=ORIENTED_EDGE ( 'NONE', *, *, #2934, .F. ) ;
#11812=CARTESIAN_POINT ( 'NONE',  ( -22.46869086674645288, 11.08405874231984001, -145.0000000000000000 ) ) ;
#11827=FACE_OUTER_BOUND ( 'NONE', #2020, .T. ) ;
#11835=DIRECTION ( 'NONE',  ( 0.000000000000000000, 1.000000000000000000, 1.177509268541832635E-16 ) ) ;
#11837=DIRECTION ( 'NONE',  ( -0.000000000000000000, 1.000000000000000000, -0.000000000000000000 ) ) ;
#11838=VECTOR ( 'NONE', #15062, 1000.000000000000000 ) ;
#11867=EDGE_CURVE ( 'NONE', #12500, #6504, #22538, .T. ) ;
#11878=DIRECTION ( 'NONE',  ( -1.000000000000000000, 0.000000000000000000, 0.000000000000000000 ) ) ;
#11909=DIRECTION ( 'NONE',  ( -0.000000000000000000, -0.000000000000000000, 1.000000000000000000 ) ) ;
#11918=LINE ( 'NONE', #2807, #15039 ) ;
#11921=EDGE_LOOP ( 'NONE', ( #19427, #19001, #9677, #16520 ) ) ;
#11933=DIRECTION ( 'NONE',  ( 0.000000000000000000, 0.000000000000000000, 1.000000000000000000 ) ) ;
#11935=VERTEX_POINT ( 'NONE', #8074 ) ;
#11936=CARTESIAN_POINT ( 'NONE',  ( 21.69904058246457268, 12.52399064369876669, -145.0000000000000000 ) ) ;
#11950=CIRCLE ( 'NONE', #9673, 5.249999999999973355 ) ;
#11952=ADVANCED_FACE ( 'NONE', ( #20868, #15456, #4553, #22661, #4438 ), #10367, .T. ) ;
#11994=DIRECTION ( 'NONE',  ( 0.000000000000000000, 1.000000000000000000, 0.000000000000000000 ) ) ;
#12046=FILL_AREA_STYLE ('',( #4626 ) ) ;
#12049=EDGE_LOOP ( 'NONE', ( #11538, #21814, #1254, #3170 ) ) ;
#12056=VERTEX_POINT ( 'NONE', #18189 ) ;
#12069=CARTESIAN_POINT ( 'NONE',  ( -6.487720808684898977, 24.19924082458020820, -145.0000000000000000 ) ) ;
#12088=DIRECTION ( 'NONE',  ( 1.000000000000000000, 0.000000000000000000, 0.000000000000000000 ) ) ;
#12109=DIRECTION ( 'NONE',  ( -0.000000000000000000, -1.177509268541832635E-16, 1.000000000000000000 ) ) ;
#12135=ORIENTED_EDGE ( 'NONE', *, *, #8582, .T. ) ;
#12146=( LENGTH_UNIT ( ) NAMED_UNIT ( * ) SI_UNIT ( .MILLI., .METRE. ) );
#12163=ORIENTED_EDGE ( 'NONE', *, *, #6326, .T. ) ;
#12204=DIRECTION ( 'NONE',  ( 0.000000000000000000, -1.000000000000000000, -1.177509268541832635E-16 ) ) ;
#12229=EDGE_LOOP ( 'NONE', ( #16304, #22224, #6707, #10699 ) ) ;
#12232=EDGE_LOOP ( 'NONE', ( #8715, #5853 ) ) ;
#12238=CARTESIAN_POINT ( 'NONE',  ( 45.00000000000000000, 269.9999999999999432, 0.000000000000000000 ) ) ;
#12240=ORIENTED_EDGE ( 'NONE', *, *, #4893, .F. ) ;
#12241=CARTESIAN_POINT ( 'NONE',  ( 72.64999999999999147, -112.6666666666666714, 144.9999999999999716 ) ) ;
#12281=DIRECTION ( 'NONE',  ( 0.000000000000000000, -1.000000000000000000, -1.110223024625156540E-16 ) ) ;
#12295=CARTESIAN_POINT ( 'NONE',  ( 0.000000000000000000, -1000.000000000000000, -138.9999999999999716 ) ) ;
#12298=CIRCLE ( 'NONE', #8410, 2.649999999999985700 ) ;
#12300=EDGE_CURVE ( 'NONE', #8946, #14733, #20945, .T. ) ;
#12311=CARTESIAN_POINT ( 'NONE',  ( 0.000000000000000000, -1000.000000000000000, 145.0000119999999697 ) ) ;
#12336=VERTEX_POINT ( 'NONE', #21067 ) ;
#12338=EDGE_CURVE ( 'NONE', #5249, #5237, #16717, .T. ) ;
#12403=AXIS2_PLACEMENT_3D ( 'NONE', #926, #6617, #23015 ) ;
#12406=ORIENTED_EDGE ( 'NONE', *, *, #9667, .T. ) ;
#12414=LINE ( 'NONE', #4644, #14197 ) ;
#12426=( LENGTH_UNIT ( ) NAMED_UNIT ( * ) SI_UNIT ( .MILLI., .METRE. ) );
#12447=CARTESIAN_POINT ( 'NONE',  ( 40.00000000000000000, 100.0000000000000000, 125.0000000000000000 ) ) ;
#12450=ORIENTED_EDGE ( 'NONE', *, *, #12685, .T. ) ;
#12471=VERTEX_POINT ( 'NONE', #20848 ) ;
#12476=EDGE_CURVE ( 'NONE', #22877, #12500, #9969, .T. ) ;
#12497=CARTESIAN_POINT ( 'NONE',  ( 24.99999999999999645, -5.982013681773172432E-16, -145.0000059999999849 ) ) ;
#12500=VERTEX_POINT ( 'NONE', #2324 ) ;
#12501=ADVANCED_FACE ( 'NONE', ( #4261 ), #4374, .F. ) ;
#12534=VECTOR ( 'NONE', #15350, 1000.000000000000000 ) ;
#12541=ORIENTED_EDGE ( 'NONE', *, *, #5727, .F. ) ;
#12604=ORIENTED_EDGE ( 'NONE', *, *, #8582, .F. ) ;
#12606=CIRCLE ( 'NONE', #13750, 20.00000000000000000 ) ;
#12621=DIRECTION ( 'NONE',  ( 0.000000000000000000, 0.000000000000000000, 1.000000000000000000 ) ) ;
#12628=EDGE_LOOP ( 'NONE', ( #14526, #18153 ) ) ;
#12633=CARTESIAN_POINT ( 'NONE',  ( 20.00000000000000000, -1000.000000000000000, 124.9999999999998579 ) ) ;
#12660=VERTEX_POINT ( 'NONE', #5561 ) ;
#12663=FACE_OUTER_BOUND ( 'NONE', #1889, .T. ) ;
#12681=FACE_BOUND ( 'NONE', #2735, .T. ) ;
#12685=EDGE_CURVE ( 'NONE', #2118, #20062, #997, .T. ) ;
#12686=CARTESIAN_POINT ( 'NONE',  ( 24.99999999999999645, 2.463415629691065208E-15, 145.0000059999999849 ) ) ;
#12692=CARTESIAN_POINT ( 'NONE',  ( -45.24999999999994316, 100.0000000000000000, -145.0000000000000284 ) ) ;
#12720=CARTESIAN_POINT ( 'NONE',  ( 15.24974479720506970, -19.87769063953885507, 145.0000119999999413 ) ) ;
#12724=EDGE_CURVE ( 'NONE', #12471, #6599, #11644, .T. ) ;
#12725=VECTOR ( 'NONE', #8658, 1000.000000000000000 ) ;
#12737=AXIS2_PLACEMENT_3D ( 'NONE', #20840, #1991, #19006 ) ;
#12738=CARTESIAN_POINT ( 'NONE',  ( 34.75000000000005684, 100.0000000000000000, 150.2000000000009550 ) ) ;
#12743=EDGE_CURVE ( 'NONE', #21577, #3347, #23667, .T. ) ;
#12745=CARTESIAN_POINT ( 'NONE',  ( -16.52066876451826616, -1018.834670294809257, 145.0000119999999981 ) ) ;
#12750=ORIENTED_EDGE ( 'NONE', *, *, #15108, .T. ) ;
#12758=CARTESIAN_POINT ( 'NONE',  ( -25.00000000000000000, 1.865214261513747767E-15, 145.0000119999999697 ) ) ;
#12769=EDGE_CURVE ( 'NONE', #12500, #22877, #15463, .T. ) ;
#12802=DIRECTION ( 'NONE',  ( 0.000000000000000000, 0.000000000000000000, -1.000000000000000000 ) ) ;
#12810=ORIENTED_EDGE ( 'NONE', *, *, #179, .F. ) ;
#12817=CARTESIAN_POINT ( 'NONE',  ( -21.69578997558840427, 12.52876685377503208, 145.0000119999999697 ) ) ;
#12841=CARTESIAN_POINT ( 'NONE',  ( 34.75000000000005684, 100.0000000000000000, -125.0000000000000000 ) ) ;
#12854=ORIENTED_EDGE ( 'NONE', *, *, #16972, .T. ) ;
#12857=CARTESIAN_POINT ( 'NONE',  ( 12.52876685377503208, -1021.695789975588241, 145.0000119999999697 ) ) ;
#12884=CARTESIAN_POINT ( 'NONE',  ( 15.25457574328937227, -980.1254780500729566, -145.0000000000001137 ) ) ;
#12901=FACE_OUTER_BOUND ( 'NONE', #19548, .T. ) ;
#12920=ORIENTED_EDGE ( 'NONE', *, *, #10932, .T. ) ;
#12947=SHAPE_DEFINITION_REPRESENTATION ( #17677, #15622 ) ;
#12949=AXIS2_PLACEMENT_3D ( 'NONE', #7638, #15032, #11189 ) ;
#12950=FACE_OUTER_BOUND ( 'NONE', #4221, .T. ) ;
#12977=DIRECTION ( 'NONE',  ( 0.000000000000000000, -1.000000000000000000, 0.000000000000000000 ) ) ;
#12978=EDGE_CURVE ( 'NONE', #22845, #13209, #20969, .T. ) ;
#13007=AXIS2_PLACEMENT_3D ( 'NONE', #23687, #3522, #3282 ) ;
#13024=CARTESIAN_POINT ( 'NONE',  ( -24.99999999999998224, -1000.000000000000000, 145.0000059999999280 ) ) ;
#13040=CARTESIAN_POINT ( 'NONE',  ( 100.0000000000000000, 249.9999999999999716, 125.0000000000000284 ) ) ;
#13052=DIRECTION ( 'NONE',  ( -0.000000000000000000, 1.000000000000000000, 0.000000000000000000 ) ) ;
#13056=DIRECTION ( 'NONE',  ( -0.000000000000000000, -0.000000000000000000, 1.000000000000000000 ) ) ;
#13069=LINE ( 'NONE', #15102, #20744 ) ;
#13073=CARTESIAN_POINT ( 'NONE',  ( 3.272451888078301785, -24.83884780301426787, 145.0000119999999697 ) ) ;
#13075=CIRCLE ( 'NONE', #11131, 25.00000000000000000 ) ;
#13083=EDGE_LOOP ( 'NONE', ( #2367, #21884, #11640, #23632 ) ) ;
#13112=AXIS2_PLACEMENT_3D ( 'NONE', #14824, #13166, #14943 ) ;
#13122=ORIENTED_EDGE ( 'NONE', *, *, #8970, .F. ) ;
#13137=AXIS2_PLACEMENT_3D ( 'NONE', #19133, #13394, #2728 ) ;
#13145=CARTESIAN_POINT ( 'NONE',  ( 100.0000000000000000, 269.9999999999999432, 125.0000000000000284 ) ) ;
#13155=CARTESIAN_POINT ( 'NONE',  ( 1.636246173744675403, -975.0000000000000000, 145.0000119999999697 ) ) ;
#13166=DIRECTION ( 'NONE',  ( 0.000000000000000000, -1.177509268541832635E-16, 1.000000000000000000 ) ) ;
#13168=EDGE_CURVE ( 'NONE', #6672, #12336, #670, .T. ) ;
#13173=CYLINDRICAL_SURFACE ( 'NONE', #11622, 5.249999999999942268 ) ;
#13180=CARTESIAN_POINT ( 'NONE',  ( 100.0000000000000000, -1400.000000000000000, -125.0000000000001705 ) ) ;
#13209=VERTEX_POINT ( 'NONE', #10476 ) ;
#13210=FACE_OUTER_BOUND ( 'NONE', #10142, .T. ) ;
#13217=DIRECTION ( 'NONE',  ( 1.000000000000000000, 0.000000000000000000, 0.000000000000000000 ) ) ;
#13218=CARTESIAN_POINT ( 'NONE',  ( 23.72315261474501469, -1008.055391459054249, 145.0000119999999697 ) ) ;
#13220=CARTESIAN_POINT ( 'NONE',  ( 24.99999999999998224, -1000.000000000000000, 145.0000059999999280 ) ) ;
#13222=FACE_OUTER_BOUND ( 'NONE', #8685, .T. ) ;
#13229=VERTEX_POINT ( 'NONE', #18270 ) ;
#13231=EDGE_CURVE ( 'NONE', #18285, #19306, #930, .T. ) ;
#13236=VERTEX_POINT ( 'NONE', #21780 ) ;
#13264=ORIENTED_EDGE ( 'NONE', *, *, #9319, .T. ) ;
#13271=CARTESIAN_POINT ( 'NONE',  ( -24.99999999999998224, -1000.000000000000000, -138.9999999999999716 ) ) ;
#13279=CARTESIAN_POINT ( 'NONE',  ( 0.000000000000000000, 1.865214261513747767E-15, 138.9999999999999716 ) ) ;
#13286=AXIS2_PLACEMENT_3D ( 'NONE', #17149, #375, #7478 ) ;
#13287=EDGE_CURVE ( 'NONE', #21638, #20769, #11377, .T. ) ;
#13296=DIRECTION ( 'NONE',  ( -1.000000000000000000, -0.000000000000000000, -0.000000000000000000 ) ) ;
#13307=VERTEX_POINT ( 'NONE', #5126 ) ;
#13327=CARTESIAN_POINT ( 'NONE',  ( 24.20041621714722879, -993.5179357872714263, 145.0000119999999413 ) ) ;
#13339=DIRECTION ( 'NONE',  ( -0.000000000000000000, -0.000000000000000000, 1.000000000000000000 ) ) ;
#13348=EDGE_CURVE ( 'NONE', #10540, #6672, #6736, .T. ) ;
#13350=CARTESIAN_POINT ( 'NONE',  ( 100.0000000000000000, 250.0000000000000000, -124.9999999999999716 ) ) ;
#13355=CARTESIAN_POINT ( 'NONE',  ( -19.87452195017631595, -984.7454242570835277, -145.0000000000001137 ) ) ;
#13357=CIRCLE ( 'NONE', #207, 5.249999999999956479 ) ;
#13361=VERTEX_POINT ( 'NONE', #11308 ) ;
#13373=EDGE_LOOP ( 'NONE', ( #17256, #10802 ) ) ;
#13380=VERTEX_POINT ( 'NONE', #5596 ) ;
#13392=EDGE_CURVE ( 'NONE', #12336, #2069, #10211, .T. ) ;
#13394=DIRECTION ( 'NONE',  ( 0.000000000000000000, 0.000000000000000000, 1.000000000000000000 ) ) ;
#13405=FACE_BOUND ( 'NONE', #18508, .T. ) ;
#13410=VERTEX_POINT ( 'NONE', #5479 ) ;
#13421=EDGE_CURVE ( 'NONE', #5237, #5249, #165, .T. ) ;
#13422=EDGE_CURVE ( 'NONE', #2021, #8380, #18654, .T. ) ;
#13442=EDGE_LOOP ( 'NONE', ( #15738, #12920, #9049, #5233 ) ) ;
#13444=FACE_OUTER_BOUND ( 'NONE', #15154, .T. ) ;
#13445=CARTESIAN_POINT ( 'NONE',  ( -21.69904058246455847, -1012.523990643698880, -145.0000000000001421 ) ) ;
#13475=AXIS2_PLACEMENT_3D ( 'NONE', #4675, #12088, #12802 ) ;
#13482=CARTESIAN_POINT ( 'NONE',  ( -23.72531794788157100, -991.9499648419341611, -145.0000000000001421 ) ) ;
#13492=EDGE_CURVE ( 'NONE', #8328, #19306, #16467, .T. ) ;
#13500=FACE_BOUND ( 'NONE', #13373, .T. ) ;
#13510=DIRECTION ( 'NONE',  ( 1.000000000000000000, 0.000000000000000000, 0.000000000000000000 ) ) ;
#13519=CARTESIAN_POINT ( 'NONE',  ( 15.25457574233253055, 19.87452195056642168, -145.0000000000000000 ) ) ;
#13520=AXIS2_PLACEMENT_3D ( 'NONE', #448, #17354, #4411 ) ;
#13531=CARTESIAN_POINT ( 'NONE',  ( 100.0000000000000000, 249.9999999999999716, 145.0000000000000284 ) ) ;
#13532=DIRECTION ( 'NONE',  ( 0.000000000000000000, 0.000000000000000000, 1.000000000000000000 ) ) ;
#13538=( GEOMETRIC_REPRESENTATION_CONTEXT ( 3 ) GLOBAL_UNCERTAINTY_ASSIGNED_CONTEXT ( ( #6007 ) ) GLOBAL_UNIT_ASSIGNED_CONTEXT ( ( #12146, #17650, #2050 ) ) REPRESENTATION_CONTEXT ( 'NONE', 'WORKASPACE' ) );
#13540=AXIS2_PLACEMENT_3D ( 'NONE', #3263, #8721, #1454 ) ;
#13541=PLANE ( 'NONE',  #9068 ) ;
#13556=CARTESIAN_POINT ( 'NONE',  ( 70.00000000000000000, -87.33333333333332860, 145.0000000000000000 ) ) ;
#13569=CARTESIAN_POINT ( 'NONE',  ( 19.87769063953886928, -15.24974479720507148, 145.0000119999999981 ) ) ;
#13584=CARTESIAN_POINT ( 'NONE',  ( 0.000000000000000000, 0.000000000000000000, -150.0000000000000000 ) ) ;
#13593=DIRECTION ( 'NONE',  ( 0.000000000000000000, 1.000000000000000000, 0.000000000000000000 ) ) ;
#13595=CARTESIAN_POINT ( 'NONE',  ( -11.08405391225051595, -22.46867509500516036, -145.0000000000000000 ) ) ;
#13596=ORIENTED_EDGE ( 'NONE', *, *, #14506, .T. ) ;
#13599=VERTEX_POINT ( 'NONE', #15624 ) ;
#13605=CARTESIAN_POINT ( 'NONE',  ( 45.24999999999994316, 100.0000000000000000, 145.0000000000000000 ) ) ;
#13627=AXIS2_PLACEMENT_3D ( 'NONE', #574, #15200, #8299 ) ;
#13632=DIRECTION ( 'NONE',  ( 0.000000000000000000, 0.000000000000000000, 1.000000000000000000 ) ) ;
#13634=CARTESIAN_POINT ( 'NONE',  ( 3.266776071704960316, 24.83992656739923177, -145.0000000000000000 ) ) ;
#13648=DIRECTION ( 'NONE',  ( 0.000000000000000000, 0.000000000000000000, 1.000000000000000000 ) ) ;
#13649=CARTESIAN_POINT ( 'NONE',  ( -40.00000000000000000, 100.0000000000000000, 150.2000000000009550 ) ) ;
#13658=DIRECTION ( 'NONE',  ( -0.000000000000000000, 1.000000000000000000, -0.000000000000000000 ) ) ;
#13703=ORIENTED_EDGE ( 'NONE', *, *, #21629, .T. ) ;
#13707=CARTESIAN_POINT ( 'NONE',  ( 20.00000000000000000, 0.000000000000000000, -150.0000000000000000 ) ) ;
#13725=ORIENTED_EDGE ( 'NONE', *, *, #13422, .T. ) ;
#13731=DIRECTION ( 'NONE',  ( -0.000000000000000000, -0.000000000000000000, 1.000000000000000000 ) ) ;
#13733=ORIENTED_EDGE ( 'NONE', *, *, #22640, .F. ) ;
#13745=CARTESIAN_POINT ( 'NONE',  ( -24.99999999999999645, 9.326071307568738836E-16, -145.0000059999999849 ) ) ;
#13750=AXIS2_PLACEMENT_3D ( 'NONE', #14963, #20725, #5779 ) ;
#13760=ORIENTED_EDGE ( 'NONE', *, *, #9057, .T. ) ;
#13774=DIRECTION ( 'NONE',  ( 0.000000000000000000, -1.177509268541832635E-16, 1.000000000000000000 ) ) ;
#13777=ORIENTED_EDGE ( 'NONE', *, *, #20857, .F. ) ;
#13785=DIRECTION ( 'NONE',  ( 1.000000000000000000, 0.000000000000000000, 0.000000000000000000 ) ) ;
#13800=LINE ( 'NONE', #21252, #19865 ) ;
#13831=AXIS2_PLACEMENT_3D ( 'NONE', #18368, #18031, #21766 ) ;
#13832=CARTESIAN_POINT ( 'NONE',  ( -8.050072859967423611, -976.2745910299377101, -145.0000000000001137 ) ) ;
#13850=VERTEX_POINT ( 'NONE', #20281 ) ;
#13862=CARTESIAN_POINT ( 'NONE',  ( -1.642023387316847050, 24.99995073929417444, -145.0000000000000000 ) ) ;
#13869=AXIS2_PLACEMENT_3D ( 'NONE', #11758, #9921, #8792 ) ;
#13886=CARTESIAN_POINT ( 'NONE',  ( 45.00000000000000000, 272.9999999999999432, 5.249999999999973355 ) ) ;
#13898=ADVANCED_FACE ( 'NONE', ( #9330, #13222 ), #16564, .T. ) ;
#13904=CARTESIAN_POINT ( 'NONE',  ( -12.52393590864752682, -1021.698958664561019, -145.0000000000001421 ) ) ;
#13919=ORIENTED_EDGE ( 'NONE', *, *, #12769, .F. ) ;
#13923=CARTESIAN_POINT ( 'NONE',  ( 45.24999999999994316, 100.0000000000000000, 150.2000000000009550 ) ) ;
#13951=CARTESIAN_POINT ( 'NONE',  ( -3.267023609986814847, -24.83987733669349751, -145.0000000000000000 ) ) ;
#13986=CARTESIAN_POINT ( 'NONE',  ( 24.99999999999999645, -5.982013681773172432E-16, -145.0000059999999849 ) ) ;
#14011=CARTESIAN_POINT ( 'NONE',  ( 11.08409875735507377, -1022.468567656124719, -145.0000000000001421 ) ) ;
#14035=ORIENTED_EDGE ( 'NONE', *, *, #2472, .F. ) ;
#14074=DIRECTION ( 'NONE',  ( -0.000000000000000000, -0.000000000000000000, 1.000000000000000000 ) ) ;
#14089=CARTESIAN_POINT ( 'NONE',  ( 100.0000000000000000, -1400.000000000000000, -125.0000000000001705 ) ) ;
#14126=CARTESIAN_POINT ( 'NONE',  ( 21.69895866468613121, -1012.523935908702356, -145.0000000000001421 ) ) ;
#14130=AXIS2_PLACEMENT_3D ( 'NONE', #6751, #6392, #15834 ) ;
#14163=ORIENTED_EDGE ( 'NONE', *, *, #19012, .T. ) ;
#14171=ORIENTED_EDGE ( 'NONE', *, *, #14981, .T. ) ;
#14193=CIRCLE ( 'NONE', #5309, 20.00000000000001776 ) ;
#14197=VECTOR ( 'NONE', #18501, 1000.000000000000000 ) ;
#14227=CARTESIAN_POINT ( 'NONE',  ( 0.000000000000000000, 1.865214261513747767E-15, -145.0000119999999697 ) ) ;
#14229=EDGE_CURVE ( 'NONE', #14733, #218, #11605, .T. ) ;
#14234=DIRECTION ( 'NONE',  ( 0.000000000000000000, 1.000000000000000000, 0.000000000000000000 ) ) ;
#14242=ORIENTED_EDGE ( 'NONE', *, *, #1472, .F. ) ;
#14243=CARTESIAN_POINT ( 'NONE',  ( 70.00000000000000000, -87.33333333333332860, 124.9999999999999858 ) ) ;
#14244=VECTOR ( 'NONE', #3932, 1000.000000000000000 ) ;
#14299=AXIS2_PLACEMENT_3D ( 'NONE', #16027, #18185, #14234 ) ;
#14315=AXIS2_PLACEMENT_3D ( 'NONE', #13279, #13532, #7807 ) ;
#14325=EDGE_CURVE ( 'NONE', #1314, #19715, #18844, .T. ) ;
#14326=DIRECTION ( 'NONE',  ( 1.000000000000000000, 0.000000000000000000, 0.000000000000000000 ) ) ;
#14353=LINE ( 'NONE', #14566, #18738 ) ;
#14372=CARTESIAN_POINT ( 'NONE',  ( 3.272451888078290683, 24.83884780301428208, 145.0000120000000265 ) ) ;
#14404=EDGE_LOOP ( 'NONE', ( #7767, #19376, #4366, #23767 ) ) ;
#14439=VECTOR ( 'NONE', #4468, 1000.000000000000000 ) ;
#14449=ORIENTED_EDGE ( 'NONE', *, *, #12685, .F. ) ;
#14453=VECTOR ( 'NONE', #19255, 1000.000000000000000 ) ;
#14454=DIRECTION ( 'NONE',  ( 1.000000000000000000, 0.000000000000000000, 0.000000000000000000 ) ) ;
#14470=CARTESIAN_POINT ( 'NONE',  ( 15.24974479720505549, 19.87769063953887283, 145.0000119999999697 ) ) ;
#14506=EDGE_CURVE ( 'NONE', #2113, #23382, #8111, .T. ) ;
#14519=EDGE_LOOP ( 'NONE', ( #12541, #20998 ) ) ;
#14521=CARTESIAN_POINT ( 'NONE',  ( -24.99999999999998224, -1001.636246173744439, 145.0000119999999697 ) ) ;
#14526=ORIENTED_EDGE ( 'NONE', *, *, #12769, .T. ) ;
#14538=CIRCLE ( 'NONE', #17604, 20.00000000000001776 ) ;
#14540=DIRECTION ( 'NONE',  ( 0.000000000000000000, 0.000000000000000000, 1.000000000000000000 ) ) ;
#14566=CARTESIAN_POINT ( 'NONE',  ( -72.64999999999996305, -112.6666666666667140, 148.0000000000000000 ) ) ;
#14573=VECTOR ( 'NONE', #13648, 1000.000000000000000 ) ;
#14577=CARTESIAN_POINT ( 'NONE',  ( 22.46869086670261950, -1011.084058742425668, -145.0000000000001137 ) ) ;
#14579=AXIS2_PLACEMENT_3D ( 'NONE', #8981, #9343, #14326 ) ;
#14580=CYLINDRICAL_SURFACE ( 'NONE', #6897, 5.249999999999942268 ) ;
#14581=CARTESIAN_POINT ( 'NONE',  ( -16.52066876451830524, 18.83467029480907584, 145.0000119999999697 ) ) ;
#14583=ORIENTED_EDGE ( 'NONE', *, *, #4904, .T. ) ;
#14584=ORIENTED_EDGE ( 'NONE', *, *, #10769, .F. ) ;
#14585=DIRECTION ( 'NONE',  ( -0.000000000000000000, -1.177509268541832635E-16, 1.000000000000000000 ) ) ;
#14590=ORIENTED_EDGE ( 'NONE', *, *, #19, .T. ) ;
#14593=CARTESIAN_POINT ( 'NONE',  ( 72.64999999999999147, -112.6666666666666714, 124.9999999999999858 ) ) ;
#14601=VERTEX_POINT ( 'NONE', #8207 ) ;
#14632=CARTESIAN_POINT ( 'NONE',  ( 0.000000000000000000, 0.000000000000000000, -150.0000000000000000 ) ) ;
#14636=VERTEX_POINT ( 'NONE', #21347 ) ;
#14640=CARTESIAN_POINT ( 'NONE',  ( -19.87769063953884441, -1015.249744797204812, 145.0000119999999981 ) ) ;
#14643=DIRECTION ( 'NONE',  ( -0.000000000000000000, -0.000000000000000000, 1.000000000000000000 ) ) ;
#14645=PRODUCT_DEFINITION ( 'UNKNOWN', '', #4237, #362 ) ;
#14650=VERTEX_POINT ( 'NONE', #1187 ) ;
#14669=VERTEX_POINT ( 'NONE', #1294 ) ;
#14678=AXIS2_PLACEMENT_3D ( 'NONE', #15234, #17039, #11878 ) ;
#14707=CARTESIAN_POINT ( 'NONE',  ( 24.19933745023729443, -1006.487655866706632, -145.0000000000001137 ) ) ;
#14710=CARTESIAN_POINT ( 'NONE',  ( -3.272451888078327098, 24.83884780301426787, 145.0000119999999697 ) ) ;
#14713=VERTEX_POINT ( 'NONE', #12692 ) ;
#14733=VERTEX_POINT ( 'NONE', #5512 ) ;
#14756=CARTESIAN_POINT ( 'NONE',  ( -1.636246173744678067, -1025.000000000000000, 145.0000119999999697 ) ) ;
#14785=AXIS2_PLACEMENT_3D ( 'NONE', #2019, #20034, #7116 ) ;
#14808=DIRECTION ( 'NONE',  ( 0.000000000000000000, -1.000000000000000000, 0.000000000000000000 ) ) ;
#14824=CARTESIAN_POINT ( 'NONE',  ( 100.0000000000000000, -1400.000000000000000, -145.0000000000001705 ) ) ;
#14826=CARTESIAN_POINT ( 'NONE',  ( -11.07878015919986581, 22.47082401081930669, 145.0000119999999697 ) ) ;
#14914=DIRECTION ( 'NONE',  ( 0.000000000000000000, 0.000000000000000000, 1.000000000000000000 ) ) ;
#14935=ADVANCED_FACE ( 'NONE', ( #17227 ), #13173, .F. ) ;
#14943=DIRECTION ( 'NONE',  ( 0.000000000000000000, -1.000000000000000000, -1.177509268541832635E-16 ) ) ;
#14949=FACE_BOUND ( 'NONE', #17183, .T. ) ;
#14952=EDGE_CURVE ( 'NONE', #4961, #12471, #18147, .T. ) ;
#14957=ORIENTED_EDGE ( 'NONE', *, *, #3434, .T. ) ;
#14963=CARTESIAN_POINT ( 'NONE',  ( 0.000000000000000000, -1000.000000000000000, 138.9999999999999716 ) ) ;
#14979=CARTESIAN_POINT ( 'NONE',  ( -8.055391459054607850, -23.72315261474502890, 145.0000119999999981 ) ) ;
#14981=EDGE_CURVE ( 'NONE', #13599, #14601, #22759, .T. ) ;
#14986=AXIS2_PLACEMENT_3D ( 'NONE', #4672, #1390, #2949 ) ;
#14997=CARTESIAN_POINT ( 'NONE',  ( 22.47082401081929603, -1011.078780159200051, 145.0000119999999697 ) ) ;
#15000=DIRECTION ( 'NONE',  ( 1.000000000000000000, 0.000000000000000000, 0.000000000000000000 ) ) ;
#15010=DIRECTION ( 'NONE',  ( 0.000000000000000000, -1.177509268541832635E-16, 1.000000000000000000 ) ) ;
#15032=DIRECTION ( 'NONE',  ( 0.000000000000000000, -1.177509268541832635E-16, 1.000000000000000000 ) ) ;
#15039=VECTOR ( 'NONE', #4509, 1000.000000000000000 ) ;
#15045=DIRECTION ( 'NONE',  ( 0.000000000000000000, 1.177509268541832635E-16, -1.000000000000000000 ) ) ;
#15062=DIRECTION ( 'NONE',  ( 0.000000000000000000, -1.110223024625156540E-16, 1.000000000000000000 ) ) ;
#15084=EDGE_CURVE ( 'NONE', #1956, #10702, #5036, .T. ) ;
#15088=CARTESIAN_POINT ( 'NONE',  ( 70.00000000000000000, -112.6666666666666714, 124.9999999999999858 ) ) ;
#15098=EDGE_LOOP ( 'NONE', ( #4614, #8198 ) ) ;
#15102=CARTESIAN_POINT ( 'NONE',  ( 100.0000000000000000, -1420.000000000000000, 144.9999999999998295 ) ) ;
#15108=EDGE_CURVE ( 'NONE', #6672, #10540, #18129, .T. ) ;
#15116=ORIENTED_EDGE ( 'NONE', *, *, #4332, .T. ) ;
#15125=CARTESIAN_POINT ( 'NONE',  ( -24.99995073929423484, -1001.642023388033635, -145.0000000000001137 ) ) ;
#15127=LINE ( 'NONE', #17044, #6919 ) ;
#15135=CARTESIAN_POINT ( 'NONE',  ( -69.99999999999997158, -112.6666666666667140, 148.0000000000000000 ) ) ;
#15151=AXIS2_PLACEMENT_3D ( 'NONE', #22788, #22531, #917 ) ;
#15154=EDGE_LOOP ( 'NONE', ( #12240, #14163, #10450, #4494 ) ) ;
#15168=CARTESIAN_POINT ( 'NONE',  ( -100.0000000000000000, -1400.000000000000000, -145.0000000000001705 ) ) ;
#15200=DIRECTION ( 'NONE',  ( -0.000000000000000000, -1.177509268541832635E-16, 1.000000000000000000 ) ) ;
#15228=EDGE_LOOP ( 'NONE', ( #3640, #10726 ) ) ;
#15234=CARTESIAN_POINT ( 'NONE',  ( 0.000000000000000000, 0.000000000000000000, -138.9999999999999716 ) ) ;
#15246=DIRECTION ( 'NONE',  ( 0.000000000000000000, 0.000000000000000000, -1.000000000000000000 ) ) ;
#15247=VERTEX_POINT ( 'NONE', #2335 ) ;
#15257=FACE_BOUND ( 'NONE', #23611, .T. ) ;
#15289=CARTESIAN_POINT ( 'NONE',  ( 0.000000000000000000, -1000.000000000000000, 138.9999999999999716 ) ) ;
#15293=DIRECTION ( 'NONE',  ( 0.000000000000000000, 0.000000000000000000, 1.000000000000000000 ) ) ;
#15330=VECTOR ( 'NONE', #8097, 1000.000000000000000 ) ;
#15335=CYLINDRICAL_SURFACE ( 'NONE', #18389, 2.649999999999985700 ) ;
#15338=EDGE_CURVE ( 'NONE', #22067, #22845, #4134, .T. ) ;
#15340=AXIS2_PLACEMENT_3D ( 'NONE', #1650, #20232, #9276 ) ;
#15350=DIRECTION ( 'NONE',  ( 0.000000000000000000, 1.000000000000000000, 1.177509268541832635E-16 ) ) ;
#15370=ORIENTED_EDGE ( 'NONE', *, *, #17309, .F. ) ;
#15381=ORIENTED_EDGE ( 'NONE', *, *, #13287, .F. ) ;
#15392=ORIENTED_EDGE ( 'NONE', *, *, #19738, .T. ) ;
#15432=CARTESIAN_POINT ( 'NONE',  ( -24.83884780301427497, 3.272451888078296012, 145.0000119999999697 ) ) ;
#15437=DIRECTION ( 'NONE',  ( -0.000000000000000000, 1.000000000000000000, -0.000000000000000000 ) ) ;
#15456=FACE_BOUND ( 'NONE', #6142, .T. ) ;
#15463=B_SPLINE_CURVE_WITH_KNOTS ( 'NONE', 3,
 ( #496, #15125, #16911, #19393, #15805, #4686, #13445, #18948, #2851, #22570, #2410, #13904, #9799, #7744, #17156, #612, #10253, #23151, #6618, #17592, #22454, #14011, #21340, #8554, #15922, #23258, #6730, #14126, #14577, #22044, #14707, #10976, #10869, #5504 ),
 .UNSPECIFIED., .F., .F.,
 ( 4, 2, 2, 2, 2, 2, 2, 2, 2, 2, 2, 2, 2, 2, 2, 2, 4 ),
 ( 0.7500000000000000000, 0.7812500000000000000, 0.8125000000000000000, 0.8437500000000000000, 0.8750000000000000000, 0.9062500000000000000, 0.9375000000000000000, 0.9687500000000000000, 1.000000000000000000, 1.031250000000000000, 1.062500000000000000, 1.093750000000000000, 1.125000000000000000, 1.156250000000000000, 1.187500000000000000, 1.218750000000000000, 1.250000000000000000 ),
 .UNSPECIFIED. ) ;
#15469=EDGE_LOOP ( 'NONE', ( #4925, #5660, #2524, #4448 ) ) ;
#15475=CYLINDRICAL_SURFACE ( 'NONE', #10371, 24.99999999999998224 ) ;
#15478=EDGE_CURVE ( 'NONE', #19715, #1956, #17433, .T. ) ;
#15498=CARTESIAN_POINT ( 'NONE',  ( -24.99995073930943690, -1.642023387880738428, -145.0000000000000284 ) ) ;
#15511=CARTESIAN_POINT ( 'NONE',  ( -3.266795291543685309, -975.1599768041793368, -145.0000000000001137 ) ) ;
#15524=CARTESIAN_POINT ( 'NONE',  ( -45.24999999999994316, 100.0000000000000000, 145.0000000000000000 ) ) ;
#15535=VERTEX_POINT ( 'NONE', #23330 ) ;
#15539=CARTESIAN_POINT ( 'NONE',  ( -3.266795292121510208, 24.84002319558113214, -145.0000000000000000 ) ) ;
#15570=DIRECTION ( 'NONE',  ( 0.000000000000000000, 1.177509268541832635E-16, -1.000000000000000000 ) ) ;
#15595=ORIENTED_EDGE ( 'NONE', *, *, #6326, .F. ) ;
#15596=VERTEX_POINT ( 'NONE', #12633 ) ;
#15598=VECTOR ( 'NONE', #9403, 1000.000000000000000 ) ;
#15610=CARTESIAN_POINT ( 'NONE',  ( 21.69892645970834621, -12.52401366503153213, -145.0000000000000000 ) ) ;
#15614=DIRECTION ( 'NONE',  ( 0.000000000000000000, 1.000000000000000000, 1.177509268541832635E-16 ) ) ;
#15620=CARTESIAN_POINT ( 'NONE',  ( -21.69895866495090786, -987.4760640919365642, -145.0000000000001421 ) ) ;
#15622=SHAPE_REPRESENTATION ( 'support structure', ( #11210 ), #16580 ) ;
#15624=CARTESIAN_POINT ( 'NONE',  ( 25.00000000000000000, 4.926831259382130415E-15, 138.9999999999999716 ) ) ;
#15628=ORIENTED_EDGE ( 'NONE', *, *, #19447, .T. ) ;
#15642=DIRECTION ( 'NONE',  ( 0.000000000000000000, 0.000000000000000000, -1.000000000000000000 ) ) ;
#15647=ORIENTED_EDGE ( 'NONE', *, *, #18589, .F. ) ;
#15659=CYLINDRICAL_SURFACE ( 'NONE', #20807, 5.249999999999942268 ) ;
#15676=CARTESIAN_POINT ( 'NONE',  ( -40.00000000000000000, 100.0000000000000000, 125.0000000000000000 ) ) ;
#15684=EDGE_CURVE ( 'NONE', #20769, #21638, #7614, .T. ) ;
#15693=AXIS2_PLACEMENT_3D ( 'NONE', #21680, #3780, #23716 ) ;
#15725=FACE_BOUND ( 'NONE', #21938, .T. ) ;
#15736=AXIS2_PLACEMENT_3D ( 'NONE', #7619, #15010, #20534 ) ;
#15738=ORIENTED_EDGE ( 'NONE', *, *, #3848, .F. ) ;
#15752=CYLINDRICAL_SURFACE ( 'NONE', #5685, 5.249999999999942268 ) ;
#15755=DIRECTION ( 'NONE',  ( 0.000000000000000000, 0.000000000000000000, -1.000000000000000000 ) ) ;
#15761=CARTESIAN_POINT ( 'NONE',  ( -100.0000000000000000, -1400.000000000000000, 124.9999999999998295 ) ) ;
#15767=EDGE_CURVE ( 'NONE', #14669, #15596, #16500, .T. ) ;
#15784=DIRECTION ( 'NONE',  ( 0.000000000000000000, 0.000000000000000000, -1.000000000000000000 ) ) ;
#15805=CARTESIAN_POINT ( 'NONE',  ( -23.72540896990115655, -1008.050072860352543, -145.0000000000001421 ) ) ;
#15809=ORIENTED_EDGE ( 'NONE', *, *, #15478, .F. ) ;
#15820=VECTOR ( 'NONE', #20688, 1000.000000000000000 ) ;
#15834=DIRECTION ( 'NONE',  ( 1.000000000000000000, 0.000000000000000000, 0.000000000000000000 ) ) ;
#15837=CIRCLE ( 'NONE', #18494, 5.249999999999949374 ) ;
#15839=ORIENTED_EDGE ( 'NONE', *, *, #1586, .F. ) ;
#15859=FACE_OUTER_BOUND ( 'NONE', #21335, .T. ) ;
#15886=ORIENTED_EDGE ( 'NONE', *, *, #22935, .T. ) ;
#15906=CARTESIAN_POINT ( 'NONE',  ( 0.000000000000000000, 1.865214261513747767E-15, -138.9999999999999716 ) ) ;
#15918=ORIENTED_EDGE ( 'NONE', *, *, #8150, .F. ) ;
#15922=CARTESIAN_POINT ( 'NONE',  ( 16.51661849037862950, -1018.838790234052340, -145.0000000000001137 ) ) ;
#15938=EDGE_CURVE ( 'NONE', #21406, #21409, #21881, .T. ) ;
#15976=EDGE_CURVE ( 'NONE', #7122, #19888, #20482, .T. ) ;
#16002=ORIENTED_EDGE ( 'NONE', *, *, #5116, .F. ) ;
#16019=VECTOR ( 'NONE', #6388, 1000.000000000000000 ) ;
#16027=CARTESIAN_POINT ( 'NONE',  ( -69.99999999999997158, -87.33333333333338544, 124.9999999999999858 ) ) ;
#16038=CYLINDRICAL_SURFACE ( 'NONE', #13869, 5.249999999999942268 ) ;
#16063=EDGE_CURVE ( 'NONE', #11935, #15535, #22781, .T. ) ;
#16101=EDGE_CURVE ( 'NONE', #17429, #22939, #11155, .T. ) ;
#16140=DIRECTION ( 'NONE',  ( 0.000000000000000000, 1.177509268541832635E-16, -1.000000000000000000 ) ) ;
#16149=ORIENTED_EDGE ( 'NONE', *, *, #3662, .F. ) ;
#16157=CARTESIAN_POINT ( 'NONE',  ( 24.20041621714724300, 6.482064212728136710, 145.0000119999999697 ) ) ;
#16171=AXIS2_PLACEMENT_3D ( 'NONE', #11126, #1907, #17482 ) ;
#16176=ORIENTED_EDGE ( 'NONE', *, *, #7335, .F. ) ;
#16181=EDGE_CURVE ( 'NONE', #2340, #218, #21137, .T. ) ;
#16239=ADVANCED_FACE ( 'NONE', ( #10232 ), #1022, .F. ) ;
#16281=ADVANCED_FACE ( 'NONE', ( #12663 ), #15475, .F. ) ;
#16290=ADVANCED_FACE ( 'NONE', ( #12901 ), #23491, .F. ) ;
#16304=ORIENTED_EDGE ( 'NONE', *, *, #2023, .F. ) ;
#16319=EDGE_LOOP ( 'NONE', ( #12450, #7068, #11426, #15370 ) ) ;
#16354=DIRECTION ( 'NONE',  ( 0.000000000000000000, -1.000000000000000000, 0.000000000000000000 ) ) ;
#16364=EDGE_LOOP ( 'NONE', ( #14957, #15116, #7036, #14242 ) ) ;
#16370=AXIS2_PLACEMENT_3D ( 'NONE', #9587, #419, #16949 ) ;
#16385=CARTESIAN_POINT ( 'NONE',  ( 8.055391459054625614, 23.72315261474502890, 145.0000119999999981 ) ) ;
#16421=CARTESIAN_POINT ( 'NONE',  ( 1.636246173744688726, -24.99999999999999289, 145.0000119999999697 ) ) ;
#16426=ORIENTED_EDGE ( 'NONE', *, *, #3202, .F. ) ;
#16428=ORIENTED_EDGE ( 'NONE', *, *, #2518, .T. ) ;
#16437=CARTESIAN_POINT ( 'NONE',  ( -21.69578997558838296, -1012.528766853774982, 145.0000119999999697 ) ) ;
#16439=CARTESIAN_POINT ( 'NONE',  ( -69.99999999999997158, -87.33333333333338544, 148.0000000000000000 ) ) ;
#16461=CARTESIAN_POINT ( 'NONE',  ( -100.0000000000000000, -1420.000000000000000, 124.9999999999998295 ) ) ;
#16467=LINE ( 'NONE', #19686, #4187 ) ;
#16471=CARTESIAN_POINT ( 'NONE',  ( -20.00000000000000000, 2.449293598294706513E-15, -150.0000000000000000 ) ) ;
#16484=EDGE_LOOP ( 'NONE', ( #20588, #5497, #19689, #9349 ) ) ;
#16488=ADVANCED_FACE ( 'NONE', ( #13500, #20819, #5726 ), #18626, .F. ) ;
#16499=CARTESIAN_POINT ( 'NONE',  ( -6.482064212728111841, 24.20041621714724656, 145.0000119999999697 ) ) ;
#16500=CIRCLE ( 'NONE', #17288, 20.00000000000001776 ) ;
#16520=ORIENTED_EDGE ( 'NONE', *, *, #13287, .T. ) ;
#16537=CARTESIAN_POINT ( 'NONE',  ( -1.636246173744679178, -24.99999999999999645, 145.0000119999999697 ) ) ;
#16559=CARTESIAN_POINT ( 'NONE',  ( -69.99999999999997158, -112.6666666666667140, 144.9999999999999716 ) ) ;
#16561=CARTESIAN_POINT ( 'NONE',  ( -24.99999999999998224, -1000.000000000000000, 145.0000059999999280 ) ) ;
#16562=FACE_OUTER_BOUND ( 'NONE', #14404, .T. ) ;
#16564=PLANE ( 'NONE',  #11633 ) ;
#16577=LINE ( 'NONE', #12758, #22732 ) ;
#16580=( GEOMETRIC_REPRESENTATION_CONTEXT ( 3 ) GLOBAL_UNCERTAINTY_ASSIGNED_CONTEXT ( ( #17123 ) ) GLOBAL_UNIT_ASSIGNED_CONTEXT ( ( #8606, #21514, #19704 ) ) REPRESENTATION_CONTEXT ( 'NONE', 'WORKASPACE' ) );
#16589=CYLINDRICAL_SURFACE ( 'NONE', #18853, 5.249999999999942268 ) ;
#16612=ORIENTED_EDGE ( 'NONE', *, *, #20627, .F. ) ;
#16622=CARTESIAN_POINT ( 'NONE',  ( -8.055391459054613179, -976.2768473852549960, 145.0000119999999697 ) ) ;
#16623=EDGE_LOOP ( 'NONE', ( #1705, #6489, #8265, #10273 ) ) ;
#16633=CARTESIAN_POINT ( 'NONE',  ( 11.07878015919986758, 22.47082401081930669, 145.0000119999999697 ) ) ;
#16657=DIRECTION ( 'NONE',  ( -1.000000000000000000, -0.000000000000000000, -0.000000000000000000 ) ) ;
#16660=CARTESIAN_POINT ( 'NONE',  ( -24.20041621714726077, -6.482064212728086972, 145.0000119999999697 ) ) ;
#16663=EDGE_CURVE ( 'NONE', #14713, #8328, #17214, .T. ) ;
#16670=EDGE_CURVE ( 'NONE', #6504, #18582, #23371, .T. ) ;
#16672=ORIENTED_EDGE ( 'NONE', *, *, #9476, .T. ) ;
#16677=EDGE_CURVE ( 'NONE', #10702, #1956, #17234, .T. ) ;
#16679=CARTESIAN_POINT ( 'NONE',  ( -8.055391459054604297, -1023.723152614744549, 145.0000119999999981 ) ) ;
#16689=ORIENTED_EDGE ( 'NONE', *, *, #4728, .F. ) ;
#16701=CARTESIAN_POINT ( 'NONE',  ( 40.00000000000000000, 100.0000000000000000, 150.2000000000009550 ) ) ;
#16710=CARTESIAN_POINT ( 'NONE',  ( 24.99995073929424194, -998.3579766121645207, -145.0000000000001137 ) ) ;
#16717=CIRCLE ( 'NONE', #22870, 5.249999999999949374 ) ;
#16728=CARTESIAN_POINT ( 'NONE',  ( -23.72315261474501824, -991.9446085409454099, 145.0000119999999697 ) ) ;
#16749=AXIS2_PLACEMENT_3D ( 'NONE', #8995, #17928, #16354 ) ;
#16770=ORIENTED_EDGE ( 'NONE', *, *, #8150, .T. ) ;
#16783=VERTEX_POINT ( 'NONE', #3750 ) ;
#16789=CARTESIAN_POINT ( 'NONE',  ( -3.272451888078288906, -1024.838847803014232, 145.0000119999999981 ) ) ;
#16799=ORIENTED_EDGE ( 'NONE', *, *, #19447, .F. ) ;
#16801=CIRCLE ( 'NONE', #6390, 2.649999999999999467 ) ;
#16824=CARTESIAN_POINT ( 'NONE',  ( -24.99999999999998224, -1000.000000000000000, 138.9999999999999716 ) ) ;
#16831=CIRCLE ( 'NONE', #4091, 20.00000000000000000 ) ;
#16841=EDGE_LOOP ( 'NONE', ( #1106, #22035, #11346, #14583 ) ) ;
#16857=FACE_BOUND ( 'NONE', #20820, .T. ) ;
#16867=ORIENTED_EDGE ( 'NONE', *, *, #16663, .F. ) ;
#16878=VERTEX_POINT ( 'NONE', #18836 ) ;
#16884=CARTESIAN_POINT ( 'NONE',  ( 72.64999999999999147, -87.33333333333332860, 148.0000000000000000 ) ) ;
#16892=AXIS2_PLACEMENT_3D ( 'NONE', #6731, #7976, #10507 ) ;
#16904=DIRECTION ( 'NONE',  ( 0.000000000000000000, 1.000000000000000000, 0.000000000000000000 ) ) ;
#16909=FACE_OUTER_BOUND ( 'NONE', #8228, .T. ) ;
#16911=CARTESIAN_POINT ( 'NONE',  ( -24.84002319585407292, -1003.266795291467361, -145.0000000000001137 ) ) ;
#16921=VECTOR ( 'NONE', #13296, 1000.000000000000000 ) ;
#16946=CARTESIAN_POINT ( 'NONE',  ( 24.84002319571782280, -996.7332047080466282, -145.0000000000001137 ) ) ;
#16949=DIRECTION ( 'NONE',  ( 0.000000000000000000, 1.000000000000000000, 0.000000000000000000 ) ) ;
#16971=CARTESIAN_POINT ( 'NONE',  ( 45.24999999999994316, 100.0000000000000000, -145.0000000000000284 ) ) ;
#16972=EDGE_CURVE ( 'NONE', #14733, #8946, #6528, .T. ) ;
#16977=AXIS2_PLACEMENT_3D ( 'NONE', #6284, #9797, #4348 ) ;
#16979=CARTESIAN_POINT ( 'NONE',  ( -11.07878015919985160, -977.5291759891805441, 145.0000119999999697 ) ) ;
#17008=DIRECTION ( 'NONE',  ( -0.000000000000000000, -1.177509268541832635E-16, 1.000000000000000000 ) ) ;
#17026=ORIENTED_EDGE ( 'NONE', *, *, #20857, .T. ) ;
#17037=VERTEX_POINT ( 'NONE', #19920 ) ;
#17039=DIRECTION ( 'NONE',  ( 0.000000000000000000, 0.000000000000000000, -1.000000000000000000 ) ) ;
#17044=CARTESIAN_POINT ( 'NONE',  ( -67.34999999999996589, -87.33333333333338544, 148.0000000000000000 ) ) ;
#17047=ORIENTED_EDGE ( 'NONE', *, *, #2075, .F. ) ;
#17100=FACE_OUTER_BOUND ( 'NONE', #20175, .T. ) ;
#17104=APPLICATION_CONTEXT ( 'automotive_design' ) ;
#17118=FACE_OUTER_BOUND ( 'NONE', #4103, .T. ) ;
#17123=UNCERTAINTY_MEASURE_WITH_UNIT (LENGTH_MEASURE( 1.000000000000000082E-05 ), #8606, 'distance_accuracy_value', 'NONE');
#17125=ORIENTED_EDGE ( 'NONE', *, *, #19012, .F. ) ;
#17149=CARTESIAN_POINT ( 'NONE',  ( -45.00000000000000000, 272.9999999999999432, 0.000000000000000000 ) ) ;
#17154=FACE_BOUND ( 'NONE', #14519, .T. ) ;
#17156=CARTESIAN_POINT ( 'NONE',  ( -6.487492490819623647, -1024.199386683467765, -145.0000000000001137 ) ) ;
#17158=CARTESIAN_POINT ( 'NONE',  ( 19.87769063953884441, -984.7502552027949605, 145.0000119999999981 ) ) ;
#17166=VECTOR ( 'NONE', #7237, 1000.000000000000000 ) ;
#17168=CIRCLE ( 'NONE', #6758, 2.649999999999985700 ) ;
#17177=AXIS2_PLACEMENT_3D ( 'NONE', #17776, #10171, #15614 ) ;
#17183=EDGE_LOOP ( 'NONE', ( #10394, #411 ) ) ;
#17184=CARTESIAN_POINT ( 'NONE',  ( 3.266776071109136481, -975.1600734326003703, -145.0000000000001421 ) ) ;
#17214=CIRCLE ( 'NONE', #8736, 5.249999999999949374 ) ;
#17224=ORIENTED_EDGE ( 'NONE', *, *, #17996, .T. ) ;
#17227=FACE_OUTER_BOUND ( 'NONE', #8506, .T. ) ;
#17234=CIRCLE ( 'NONE', #642, 5.249999999999949374 ) ;
#17236=EDGE_CURVE ( 'NONE', #1487, #13599, #9313, .T. ) ;
#17241=CARTESIAN_POINT ( 'NONE',  ( -25.00000000000000000, 1.865214261513747767E-15, -145.0000119999999697 ) ) ;
#17256=ORIENTED_EDGE ( 'NONE', *, *, #17960, .T. ) ;
#17264=LINE ( 'NONE', #710, #15330 ) ;
#17265=ORIENTED_EDGE ( 'NONE', *, *, #11557, .T. ) ;
#17280=CARTESIAN_POINT ( 'NONE',  ( 12.52876685377501964, -978.3042100244117592, 145.0000119999999981 ) ) ;
#17288=AXIS2_PLACEMENT_3D ( 'NONE', #22706, #5064, #13593 ) ;
#17309=EDGE_CURVE ( 'NONE', #2118, #21406, #17264, .T. ) ;
#17341=CARTESIAN_POINT ( 'NONE',  ( 11.08413645907697287, 22.46865867799474259, -145.0000000000000000 ) ) ;
#17347=AXIS2_PLACEMENT_3D ( 'NONE', #15676, #4677, #575 ) ;
#17354=DIRECTION ( 'NONE',  ( -0.000000000000000000, -1.177509268541832635E-16, 1.000000000000000000 ) ) ;
#17374=LINE ( 'NONE', #20602, #8449 ) ;
#17386=VERTEX_POINT ( 'NONE', #14593 ) ;
#17413=CARTESIAN_POINT ( 'NONE',  ( 15.25452100752526086, -19.87444003240334922, -145.0000000000000000 ) ) ;
#17424=CARTESIAN_POINT ( 'NONE',  ( 11.08413646075608305, -977.5313413224575925, -145.0000000000001137 ) ) ;
#17429=VERTEX_POINT ( 'NONE', #17742 ) ;
#17433=LINE ( 'NONE', #6316, #2326 ) ;
#17439=ORIENTED_EDGE ( 'NONE', *, *, #18589, .T. ) ;
#17443=CARTESIAN_POINT ( 'NONE',  ( 25.00000000000000000, -1.196402736354634486E-15, -138.9999999999999716 ) ) ;
#17452=CARTESIAN_POINT ( 'NONE',  ( 24.99995073930944045, 1.642023387880738428, -145.0000000000000284 ) ) ;
#17471=FACE_OUTER_BOUND ( 'NONE', #16484, .T. ) ;
#17473=CYLINDRICAL_SURFACE ( 'NONE', #15151, 2.649999999999985700 ) ;
#17474=DIRECTION ( 'NONE',  ( 0.000000000000000000, 0.000000000000000000, 1.000000000000000000 ) ) ;
#17482=DIRECTION ( 'NONE',  ( 1.000000000000000000, 0.000000000000000000, 0.000000000000000000 ) ) ;
#17491=ORIENTED_EDGE ( 'NONE', *, *, #17236, .T. ) ;
#17506=VERTEX_POINT ( 'NONE', #17855 ) ;
#17532=SURFACE_SIDE_STYLE ('',( #10188 ) ) ;
#17555=DIRECTION ( 'NONE',  ( -1.000000000000000000, -0.000000000000000000, -0.000000000000000000 ) ) ;
#17557=CARTESIAN_POINT ( 'NONE',  ( 16.51654882469418695, 18.83872056949901008, -145.0000000000000000 ) ) ;
#17560=EDGE_CURVE ( 'NONE', #20258, #21638, #2454, .T. ) ;
#17586=ADVANCED_FACE ( 'NONE', ( #8156 ), #20822, .F. ) ;
#17592=CARTESIAN_POINT ( 'NONE',  ( 6.487720807613236218, -1024.199240824787012, -145.0000000000001421 ) ) ;
#17604=AXIS2_PLACEMENT_3D ( 'NONE', #20824, #7784, #14808 ) ;
#17616=ORIENTED_EDGE ( 'NONE', *, *, #10885, .T. ) ;
#17626=ORIENTED_EDGE ( 'NONE', *, *, #9723, .F. ) ;
#17630=CARTESIAN_POINT ( 'NONE',  ( 22.46869086673244809, -11.08405874239030275, -145.0000000000000000 ) ) ;
#17638=ORIENTED_EDGE ( 'NONE', *, *, #19638, .T. ) ;
#17650=( NAMED_UNIT ( * ) PLANE_ANGLE_UNIT ( ) SI_UNIT ( $, .RADIAN. ) );
#17667=ORIENTED_EDGE ( 'NONE', *, *, #7335, .T. ) ;
#17677=PRODUCT_DEFINITION_SHAPE ( 'NONE', 'NONE',  #14645 ) ;
#17710=ORIENTED_EDGE ( 'NONE', *, *, #16063, .F. ) ;
#17715=VERTEX_POINT ( 'NONE', #23098 ) ;
#17719=CARTESIAN_POINT ( 'NONE',  ( 45.00000000000000000, 250.0000000000000000, 0.000000000000000000 ) ) ;
#17741=ADVANCED_FACE ( 'NONE', ( #8376 ), #15752, .F. ) ;
#17742=CARTESIAN_POINT ( 'NONE',  ( 20.00000000000000000, 0.000000000000000000, 124.9999999999999716 ) ) ;
#17755=CARTESIAN_POINT ( 'NONE',  ( 70.00000000000000000, -112.6666666666666714, 148.0000000000000000 ) ) ;
#17776=CARTESIAN_POINT ( 'NONE',  ( 100.0000000000000000, 249.9999999999999716, 125.0000000000000284 ) ) ;
#17780=CARTESIAN_POINT ( 'NONE',  ( 100.0000000000000000, 249.9999999999999716, 145.0000000000000284 ) ) ;
#17820=CARTESIAN_POINT ( 'NONE',  ( -40.00000000000000000, 100.0000000000000000, 145.0000000000000000 ) ) ;
#17832=CARTESIAN_POINT ( 'NONE',  ( 40.00000000000000000, 100.0000000000000000, -145.0000000000000284 ) ) ;
#17835=EDGE_CURVE ( 'NONE', #8946, #2340, #12414, .T. ) ;
#17848=DIRECTION ( 'NONE',  ( 0.000000000000000000, 1.177509268541832635E-16, -1.000000000000000000 ) ) ;
#17850=ORIENTED_EDGE ( 'NONE', *, *, #13348, .T. ) ;
#17855=CARTESIAN_POINT ( 'NONE',  ( -24.99999999999999645, -2.129009867111508370E-15, 145.0000059999999849 ) ) ;
#17871=ADVANCED_FACE ( 'NONE', ( #1823 ), #9223, .F. ) ;
#17880=CARTESIAN_POINT ( 'NONE',  ( 24.83992656990903569, -3.266860234290754672, -145.0000000000000000 ) ) ;
#17886=VECTOR ( 'NONE', #19513, 1000.000000000000000 ) ;
#17888=ORIENTED_EDGE ( 'NONE', *, *, #10932, .F. ) ;
#17891=DIRECTION ( 'NONE',  ( -1.000000000000000000, 0.000000000000000000, 0.000000000000000000 ) ) ;
#17901=ADVANCED_FACE ( 'NONE', ( #8872 ), #5466, .F. ) ;
#17928=DIRECTION ( 'NONE',  ( 0.000000000000000000, -1.177509268541832635E-16, 1.000000000000000000 ) ) ;
#17943=AXIS2_PLACEMENT_3D ( 'NONE', #77, #193, #11439 ) ;
#17960=EDGE_CURVE ( 'NONE', #12056, #6599, #8005, .T. ) ;
#17984=ORIENTED_EDGE ( 'NONE', *, *, #22640, .T. ) ;
#17996=EDGE_CURVE ( 'NONE', #14601, #13599, #13075, .T. ) ;
#18031=DIRECTION ( 'NONE',  ( -0.000000000000000000, -0.000000000000000000, 1.000000000000000000 ) ) ;
#18042=LINE ( 'NONE', #14089, #19114 ) ;
#18068=DIRECTION ( 'NONE',  ( 0.000000000000000000, -1.000000000000000000, -1.110223024625156540E-16 ) ) ;
#18072=ORIENTED_EDGE ( 'NONE', *, *, #4728, .T. ) ;
#18082=CARTESIAN_POINT ( 'NONE',  ( 23.72315261474502179, 8.055391459054641601, 145.0000119999999697 ) ) ;
#18093=CIRCLE ( 'NONE', #20377, 5.249999999999949374 ) ;
#18110=ADVANCED_FACE ( 'NONE', ( #15257, #19325, #10293, #8234, #3014, #15725, #15859, #4841, #10429 ), #2786, .T. ) ;
#18129=CIRCLE ( 'NONE', #2715, 20.00000000000000000 ) ;
#18147=CIRCLE ( 'NONE', #19291, 5.249999999999956479 ) ;
#18153=ORIENTED_EDGE ( 'NONE', *, *, #12476, .T. ) ;
#18185=DIRECTION ( 'NONE',  ( -0.000000000000000000, -1.177509268541832635E-16, 1.000000000000000000 ) ) ;
#18189=CARTESIAN_POINT ( 'NONE',  ( -45.00000000000000000, 269.9999999999999432, 5.249999999999973355 ) ) ;
#18200=FACE_OUTER_BOUND ( 'NONE', #9837, .T. ) ;
#18211=CARTESIAN_POINT ( 'NONE',  ( 100.0000000000000000, -1420.000000000000000, 124.9999999999998295 ) ) ;
#18234=EDGE_LOOP ( 'NONE', ( #18361, #18529 ) ) ;
#18236=CARTESIAN_POINT ( 'NONE',  ( 19.87769063953884796, -1015.249744797204698, 145.0000119999999697 ) ) ;
#18270=CARTESIAN_POINT ( 'NONE',  ( -72.64999999999996305, -87.33333333333338544, 145.0000000000000000 ) ) ;
#18282=CARTESIAN_POINT ( 'NONE',  ( 67.35000000000002274, -112.6666666666666714, 144.9999999999999716 ) ) ;
#18285=VERTEX_POINT ( 'NONE', #702 ) ;
#18286=CARTESIAN_POINT ( 'NONE',  ( -19.87769063953885507, -984.7502552027950742, 145.0000119999999697 ) ) ;
#18297=PLANE ( 'NONE',  #13112 ) ;
#18300=CARTESIAN_POINT ( 'NONE',  ( -1.636246173744691390, 25.00000000000000355, 145.0000119999999697 ) ) ;
#18301=ORIENTED_EDGE ( 'NONE', *, *, #14952, .F. ) ;
#18302=ORIENTED_EDGE ( 'NONE', *, *, #3725, .T. ) ;
#18309=DIRECTION ( 'NONE',  ( 0.000000000000000000, 0.000000000000000000, 1.000000000000000000 ) ) ;
#18333=LINE ( 'NONE', #16884, #8988 ) ;
#18335=CARTESIAN_POINT ( 'NONE',  ( -16.52066876451827326, -18.83467029480909005, 145.0000119999999697 ) ) ;
#18353=CARTESIAN_POINT ( 'NONE',  ( 0.000000000000000000, 1.865214261513747767E-15, -145.0000119999999697 ) ) ;
#18354=CARTESIAN_POINT ( 'NONE',  ( 20.00000000000000000, -1000.000000000000000, -138.9999999999999716 ) ) ;
#18356=DIRECTION ( 'NONE',  ( 1.000000000000000000, 0.000000000000000000, -0.000000000000000000 ) ) ;
#18361=ORIENTED_EDGE ( 'NONE', *, *, #14952, .T. ) ;
#18368=CARTESIAN_POINT ( 'NONE',  ( -69.99999999999997158, -112.6666666666667140, 148.0000000000000000 ) ) ;
#18376=EDGE_LOOP ( 'NONE', ( #23218, #4072, #1466, #5632 ) ) ;
#18389=AXIS2_PLACEMENT_3D ( 'NONE', #18679, #9532, #13785 ) ;
#18392=DIRECTION ( 'NONE',  ( -1.000000000000000000, 0.000000000000000000, 0.000000000000000000 ) ) ;
#18401=CARTESIAN_POINT ( 'NONE',  ( -100.0000000000000000, 249.9999999999999716, 125.0000000000000284 ) ) ;
#18415=ORIENTED_EDGE ( 'NONE', *, *, #4893, .T. ) ;
#18417=CYLINDRICAL_SURFACE ( 'NONE', #15340, 25.00000000000000000 ) ;
#18420=ORIENTED_EDGE ( 'NONE', *, *, #7429, .T. ) ;
#18426=EDGE_CURVE ( 'NONE', #17715, #21835, #12606, .T. ) ;
#18430=CARTESIAN_POINT ( 'NONE',  ( -45.00000000000000000, 250.0000000000000000, 0.000000000000000000 ) ) ;
#18447=EDGE_LOOP ( 'NONE', ( #16867, #6220, #19319, #6032 ) ) ;
#18450=AXIS2_PLACEMENT_3D ( 'NONE', #3053, #12281, #19352 ) ;
#18462=EDGE_CURVE ( 'NONE', #21409, #21406, #3651, .T. ) ;
#18479=CARTESIAN_POINT ( 'NONE',  ( -11.07878015919983916, -1022.470824010819570, 145.0000119999999697 ) ) ;
#18487=ORIENTED_EDGE ( 'NONE', *, *, #6202, .F. ) ;
#18494=AXIS2_PLACEMENT_3D ( 'NONE', #20815, #15045, #20925 ) ;
#18501=DIRECTION ( 'NONE',  ( 0.000000000000000000, 0.000000000000000000, 1.000000000000000000 ) ) ;
#18508=EDGE_LOOP ( 'NONE', ( #17047, #79 ) ) ;
#18529=ORIENTED_EDGE ( 'NONE', *, *, #1586, .T. ) ;
#18577=EDGE_CURVE ( 'NONE', #22067, #3718, #6401, .T. ) ;
#18582=VERTEX_POINT ( 'NONE', #4549 ) ;
#18587=CARTESIAN_POINT ( 'NONE',  ( 67.35000000000002274, -87.33333333333332860, 148.0000000000000000 ) ) ;
#18589=EDGE_CURVE ( 'NONE', #13209, #22845, #21425, .T. ) ;
#18617=CARTESIAN_POINT ( 'NONE',  ( 20.00000000000000000, -1000.000000000000000, 138.9999999999999716 ) ) ;
#18626=PLANE ( 'NONE',  #2151 ) ;
#18627=CARTESIAN_POINT ( 'NONE',  ( -20.00000000000000000, -1000.000000000000000, -125.0000000000001137 ) ) ;
#18630=AXIS2_PLACEMENT_3D ( 'NONE', #17755, #8327, #1202 ) ;
#18634=CARTESIAN_POINT ( 'NONE',  ( -67.34999999999996589, -112.6666666666667140, 124.9999999999999858 ) ) ;
#18654=CIRCLE ( 'NONE', #16370, 2.649999999999985700 ) ;
#18677=EDGE_LOOP ( 'NONE', ( #18072, #5552 ) ) ;
#18679=CARTESIAN_POINT ( 'NONE',  ( 70.00000000000000000, -87.33333333333332860, 148.0000000000000000 ) ) ;
#18698=AXIS2_PLACEMENT_3D ( 'NONE', #20977, #9653, #4435 ) ;
#18699=CARTESIAN_POINT ( 'NONE',  ( 3.272451888078299564, -1024.838847803014232, 145.0000119999999697 ) ) ;
#18712=CYLINDRICAL_SURFACE ( 'NONE', #19269, 2.649999999999999467 ) ;
#18718=ORIENTED_EDGE ( 'NONE', *, *, #15938, .T. ) ;
#18726=PLANE ( 'NONE',  #10675 ) ;
#18735=VERTEX_POINT ( 'NONE', #18401 ) ;
#18738=VECTOR ( 'NONE', #1736, 1000.000000000000000 ) ;
#18764=CARTESIAN_POINT ( 'NONE',  ( -40.00000000000000000, 100.0000000000000000, 150.2000000000009550 ) ) ;
#18765=AXIS2_PLACEMENT_3D ( 'NONE', #8765, #10593, #12977 ) ;
#18800=CARTESIAN_POINT ( 'NONE',  ( 24.83884780301427853, -3.272451888078305782, 145.0000119999999697 ) ) ;
#18820=DIRECTION ( 'NONE',  ( 0.000000000000000000, 0.000000000000000000, 1.000000000000000000 ) ) ;
#18821=CIRCLE ( 'NONE', #2632, 5.249999999999973355 ) ;
#18836=CARTESIAN_POINT ( 'NONE',  ( 67.35000000000002274, -87.33333333333332860, 145.0000000000000000 ) ) ;
#18844=CIRCLE ( 'NONE', #17347, 5.249999999999949374 ) ;
#18853=AXIS2_PLACEMENT_3D ( 'NONE', #16701, #1957, #2067 ) ;
#18858=CARTESIAN_POINT ( 'NONE',  ( 100.0000000000000000, 249.9999999999999716, 125.0000000000000284 ) ) ;
#18860=ORIENTED_EDGE ( 'NONE', *, *, #940, .F. ) ;
#18935=EDGE_CURVE ( 'NONE', #5442, #18735, #20833, .T. ) ;
#18948=CARTESIAN_POINT ( 'NONE',  ( -19.87444003266269021, -1015.254521007281141, -145.0000000000001421 ) ) ;
#18950=CARTESIAN_POINT ( 'NONE',  ( 21.69578997558837585, -987.4712331462250177, 145.0000119999999697 ) ) ;
#18988=DIRECTION ( 'NONE',  ( 0.000000000000000000, 1.110223024625156540E-16, -1.000000000000000000 ) ) ;
#19001=ORIENTED_EDGE ( 'NONE', *, *, #21833, .T. ) ;
#19006=DIRECTION ( 'NONE',  ( 1.000000000000000000, 0.000000000000000000, 0.000000000000000000 ) ) ;
#19012=EDGE_CURVE ( 'NONE', #22939, #17429, #19267, .T. ) ;
#19021=DIRECTION ( 'NONE',  ( 0.000000000000000000, 0.000000000000000000, 1.000000000000000000 ) ) ;
#19058=ADVANCED_FACE ( 'NONE', ( #2582 ), #888, .F. ) ;
#19081=EDGE_LOOP ( 'NONE', ( #3698, #18487 ) ) ;
#19113=ORIENTED_EDGE ( 'NONE', *, *, #5493, .T. ) ;
#19114=VECTOR ( 'NONE', #17555, 1000.000000000000000 ) ;
#19133=CARTESIAN_POINT ( 'NONE',  ( 0.000000000000000000, -1000.000000000000000, -150.0000000000000000 ) ) ;
#19148=ORIENTED_EDGE ( 'NONE', *, *, #15767, .T. ) ;
#19167=CARTESIAN_POINT ( 'NONE',  ( 24.99999999999999645, 2.463415629691065208E-15, 145.0000059999999849 ) ) ;
#19173=CYLINDRICAL_SURFACE ( 'NONE', #9874, 25.00000000000000000 ) ;
#19175=ORIENTED_EDGE ( 'NONE', *, *, #16670, .F. ) ;
#19180=ORIENTED_EDGE ( 'NONE', *, *, #6987, .T. ) ;
#19184=ORIENTED_EDGE ( 'NONE', *, *, #13392, .F. ) ;
#19217=DIRECTION ( 'NONE',  ( 1.000000000000000000, 0.000000000000000000, 0.000000000000000000 ) ) ;
#19242=VECTOR ( 'NONE', #11186, 1000.000000000000000 ) ;
#19249=CARTESIAN_POINT ( 'NONE',  ( 18.83879023463320124, 16.51661848982829284, -145.0000000000000000 ) ) ;
#19255=DIRECTION ( 'NONE',  ( 0.000000000000000000, 0.000000000000000000, 1.000000000000000000 ) ) ;
#19267=CIRCLE ( 'NONE', #5788, 20.00000000000000000 ) ;
#19269=AXIS2_PLACEMENT_3D ( 'NONE', #15135, #13339, #20651 ) ;
#19291=AXIS2_PLACEMENT_3D ( 'NONE', #7683, #15437, #563 ) ;
#19306=VERTEX_POINT ( 'NONE', #2290 ) ;
#19319=ORIENTED_EDGE ( 'NONE', *, *, #13231, .T. ) ;
#19321=CARTESIAN_POINT ( 'NONE',  ( 8.050072860924167628, -23.72540896942268773, -145.0000000000000000 ) ) ;
#19325=FACE_BOUND ( 'NONE', #8465, .T. ) ;
#19351=ADVANCED_BREP_SHAPE_REPRESENTATION ( '', ( #20017, #11210 ), #16580 ) ;
#19352=DIRECTION ( 'NONE',  ( 0.000000000000000000, 1.110223024625156540E-16, -1.000000000000000000 ) ) ;
#19358=ORIENTED_EDGE ( 'NONE', *, *, #19738, .F. ) ;
#19364=CARTESIAN_POINT ( 'NONE',  ( -18.83866108947328755, 16.51660830833442262, -145.0000000000000000 ) ) ;
#19376=ORIENTED_EDGE ( 'NONE', *, *, #16972, .F. ) ;
#19393=CARTESIAN_POINT ( 'NONE',  ( -24.19924082430739887, -1006.487720809339407, -145.0000000000000568 ) ) ;
#19423=ORIENTED_EDGE ( 'NONE', *, *, #14325, .F. ) ;
#19426=EDGE_LOOP ( 'NONE', ( #903, #13122, #5683, #2879 ) ) ;
#19427=ORIENTED_EDGE ( 'NONE', *, *, #9319, .F. ) ;
#19429=CARTESIAN_POINT ( 'NONE',  ( 19.87455415541893444, -15.25449798594880058, -145.0000000000000000 ) ) ;
#19447=EDGE_CURVE ( 'NONE', #7773, #4083, #108, .T. ) ;
#19465=LINE ( 'NONE', #2921, #21001 ) ;
#19513=DIRECTION ( 'NONE',  ( -0.000000000000000000, 1.000000000000000000, -0.000000000000000000 ) ) ;
#19518=ORIENTED_EDGE ( 'NONE', *, *, #12743, .F. ) ;
#19528=CARTESIAN_POINT ( 'NONE',  ( -69.99999999999997158, -87.33333333333338544, 124.9999999999999858 ) ) ;
#19548=EDGE_LOOP ( 'NONE', ( #9530, #13264, #7432, #23574 ) ) ;
#19558=CARTESIAN_POINT ( 'NONE',  ( 100.0000000000000000, -1400.000000000000000, 124.9999999999998295 ) ) ;
#19564=CARTESIAN_POINT ( 'NONE',  ( -45.00000000000000000, 269.9999999999999432, -5.249999999999973355 ) ) ;
#19602=DIRECTION ( 'NONE',  ( 0.000000000000000000, 0.000000000000000000, -1.000000000000000000 ) ) ;
#19613=ORIENTED_EDGE ( 'NONE', *, *, #431, .T. ) ;
#19623=VECTOR ( 'NONE', #20114, 1000.000000000000000 ) ;
#19637=CARTESIAN_POINT ( 'NONE',  ( -20.00000000000000000, 2.449293598294706513E-15, -138.9999999999999716 ) ) ;
#19638=EDGE_CURVE ( 'NONE', #16878, #4420, #6891, .T. ) ;
#19648=VECTOR ( 'NONE', #224, 1000.000000000000000 ) ;
#19686=CARTESIAN_POINT ( 'NONE',  ( -34.75000000000005684, 100.0000000000000000, 150.2000000000009550 ) ) ;
#19689=ORIENTED_EDGE ( 'NONE', *, *, #4493, .T. ) ;
#19700=ADVANCED_FACE ( 'NONE', ( #21583 ), #23383, .T. ) ;
#19704=( NAMED_UNIT ( * ) SI_UNIT ( $, .STERADIAN. ) SOLID_ANGLE_UNIT ( ) );
#19715=VERTEX_POINT ( 'NONE', #3100 ) ;
#19729=DIRECTION ( 'NONE',  ( 0.000000000000000000, -1.000000000000000000, 0.000000000000000000 ) ) ;
#19730=DIRECTION ( 'NONE',  ( 0.000000000000000000, 1.177509268541832635E-16, -1.000000000000000000 ) ) ;
#19738=EDGE_CURVE ( 'NONE', #14650, #13361, #9591, .T. ) ;
#19754=DIRECTION ( 'NONE',  ( 0.000000000000000000, 1.000000000000000000, 0.000000000000000000 ) ) ;
#19757=CARTESIAN_POINT ( 'NONE',  ( -20.00000000000000000, -1000.000000000000000, -150.0000000000000000 ) ) ;
#19773=VERTEX_POINT ( 'NONE', #19637 ) ;
#19783=CARTESIAN_POINT ( 'NONE',  ( 45.00000000000000000, 250.0000000000000000, 0.000000000000000000 ) ) ;
#19839=CARTESIAN_POINT ( 'NONE',  ( 24.99999999999998224, -1000.000000000000000, -145.0000119999999697 ) ) ;
#19840=CARTESIAN_POINT ( 'NONE',  ( 20.00000000000000000, 0.000000000000000000, 138.9999999999999716 ) ) ;
#19843=ORIENTED_EDGE ( 'NONE', *, *, #19, .F. ) ;
#19865=VECTOR ( 'NONE', #8572, 1000.000000000000000 ) ;
#19888=VERTEX_POINT ( 'NONE', #2587 ) ;
#19920=CARTESIAN_POINT ( 'NONE',  ( -100.0000000000000000, 270.0000000000000000, -144.9999999999999716 ) ) ;
#19953=CIRCLE ( 'NONE', #21121, 20.00000000000000000 ) ;
#19976=CARTESIAN_POINT ( 'NONE',  ( 0.000000000000000000, -1000.000000000000000, -145.0000119999999697 ) ) ;
#19978=CARTESIAN_POINT ( 'NONE',  ( 0.000000000000000000, -1000.000000000000000, -138.9999999999999716 ) ) ;
#19997=CARTESIAN_POINT ( 'NONE',  ( 12.52876685377502675, 21.69578997558840427, 145.0000119999999981 ) ) ;
#20011=DIRECTION ( 'NONE',  ( 0.000000000000000000, -1.000000000000000000, 0.000000000000000000 ) ) ;
#20017=MANIFOLD_SOLID_BREP ( 'M5 Clearance Hole1', #589 ) ;
#20034=DIRECTION ( 'NONE',  ( 0.000000000000000000, 1.177509268541832635E-16, -1.000000000000000000 ) ) ;
#20035=AXIS2_PLACEMENT_3D ( 'NONE', #22499, #657, #22855 ) ;
#20039=CARTESIAN_POINT ( 'NONE',  ( 16.52066876451828392, -18.83467029480908295, 145.0000119999999697 ) ) ;
#20045=AXIS2_PLACEMENT_3D ( 'NONE', #10248, #21097, #8551 ) ;
#20057=CARTESIAN_POINT ( 'NONE',  ( 16.52066876451827326, -1018.834670294808802, 145.0000119999999697 ) ) ;
#20062=VERTEX_POINT ( 'NONE', #4525 ) ;
#20065=SHAPE_REPRESENTATION_RELATIONSHIP ( 'NONE' , 'NONE' ,  #15622, #19351 ) ;
#20076=DIRECTION ( 'NONE',  ( 0.000000000000000000, -1.177509268541832635E-16, 1.000000000000000000 ) ) ;
#20088=CARTESIAN_POINT ( 'NONE',  ( 24.19924082444365254, -993.5122791911473996, -145.0000000000000568 ) ) ;
#20108=CARTESIAN_POINT ( 'NONE',  ( -24.83884780301426076, -996.7275481119216920, 145.0000119999999697 ) ) ;
#20114=DIRECTION ( 'NONE',  ( 0.000000000000000000, 0.000000000000000000, 1.000000000000000000 ) ) ;
#20116=FACE_BOUND ( 'NONE', #12628, .T. ) ;
#20128=CYLINDRICAL_SURFACE ( 'NONE', #2861, 24.99999999999998224 ) ;
#20132=DIRECTION ( 'NONE',  ( 0.000000000000000000, -0.000000000000000000, 1.000000000000000000 ) ) ;
#20133=LINE ( 'NONE', #13886, #8588 ) ;
#20148=CARTESIAN_POINT ( 'NONE',  ( -23.72315261474503245, -8.055391459054616732, 145.0000119999999697 ) ) ;
#20170=EDGE_LOOP ( 'NONE', ( #19518, #5823, #13733, #10317 ) ) ;
#20175=EDGE_LOOP ( 'NONE', ( #20515, #15918, #11104, #17439 ) ) ;
#20189=CARTESIAN_POINT ( 'NONE',  ( 21.69904058241862543, -987.4760093562550765, -145.0000000000001421 ) ) ;
#20206=DIRECTION ( 'NONE',  ( 0.000000000000000000, 0.000000000000000000, 1.000000000000000000 ) ) ;
#20213=CARTESIAN_POINT ( 'NONE',  ( -16.52066876451829458, -981.1653297051910840, 145.0000119999999697 ) ) ;
#20228=CARTESIAN_POINT ( 'NONE',  ( 24.83884780301427142, 3.272451888078352855, 145.0000119999999981 ) ) ;
#20232=DIRECTION ( 'NONE',  ( 0.000000000000000000, 0.000000000000000000, -1.000000000000000000 ) ) ;
#20254=CIRCLE ( 'NONE', #17943, 2.649999999999999467 ) ;
#20258=VERTEX_POINT ( 'NONE', #22726 ) ;
#20259=EDGE_CURVE ( 'NONE', #4691, #13380, #20917, .T. ) ;
#20277=CARTESIAN_POINT ( 'NONE',  ( 6.482064212728083419, -1024.200416217147222, 145.0000119999999697 ) ) ;
#20281=CARTESIAN_POINT ( 'NONE',  ( -20.00000000000000000, 2.449293598294706513E-15, 138.9999999999999716 ) ) ;
#20295=CARTESIAN_POINT ( 'NONE',  ( -45.00000000000000000, 269.9999999999999432, 0.000000000000000000 ) ) ;
#20301=ORIENTED_EDGE ( 'NONE', *, *, #12724, .F. ) ;
#20377=AXIS2_PLACEMENT_3D ( 'NONE', #11225, #8924, #23624 ) ;
#20400=EDGE_LOOP ( 'NONE', ( #14449, #17888 ) ) ;
#20413=ORIENTED_EDGE ( 'NONE', *, *, #4638, .T. ) ;
#20452=DIRECTION ( 'NONE',  ( 0.000000000000000000, -1.000000000000000000, -1.110223024625156540E-16 ) ) ;
#20459=EDGE_LOOP ( 'NONE', ( #2260, #18415, #20751, #18860 ) ) ;
#20460=CARTESIAN_POINT ( 'NONE',  ( -21.69578997558839006, -987.4712331462251313, 145.0000119999999697 ) ) ;
#20475=APPLICATION_CONTEXT ( 'automotive_design' ) ;
#20476=ORIENTED_EDGE ( 'NONE', *, *, #7429, .F. ) ;
#20482=LINE ( 'NONE', #5763, #14244 ) ;
#20498=ADVANCED_FACE ( 'NONE', ( #16562 ), #5327, .F. ) ;
#20502=EDGE_LOOP ( 'NONE', ( #22206, #20413 ) ) ;
#20503=ORIENTED_EDGE ( 'NONE', *, *, #2934, .T. ) ;
#20504=CARTESIAN_POINT ( 'NONE',  ( 12.52876685377503918, -21.69578997558838651, 145.0000119999999697 ) ) ;
#20510=CYLINDRICAL_SURFACE ( 'NONE', #11413, 5.249999999999973355 ) ;
#20514=DIRECTION ( 'NONE',  ( -0.000000000000000000, -1.177509268541832635E-16, 1.000000000000000000 ) ) ;
#20515=ORIENTED_EDGE ( 'NONE', *, *, #15338, .F. ) ;
#20519=CARTESIAN_POINT ( 'NONE',  ( 24.20041621714723590, -1006.482064212728119, 145.0000119999999697 ) ) ;
#20531=ORIENTED_EDGE ( 'NONE', *, *, #21929, .F. ) ;
#20533=FACE_OUTER_BOUND ( 'NONE', #9317, .T. ) ;
#20534=DIRECTION ( 'NONE',  ( 0.000000000000000000, -1.000000000000000000, 0.000000000000000000 ) ) ;
#20546=FACE_OUTER_BOUND ( 'NONE', #54, .T. ) ;
#20583=CARTESIAN_POINT ( 'NONE',  ( -72.64999999999996305, -112.6666666666667140, 144.9999999999999716 ) ) ;
#20587=DIRECTION ( 'NONE',  ( 1.000000000000000000, 0.000000000000000000, 0.000000000000000000 ) ) ;
#20588=ORIENTED_EDGE ( 'NONE', *, *, #179, .T. ) ;
#20594=CIRCLE ( 'NONE', #4010, 5.249999999999949374 ) ;
#20600=VERTEX_POINT ( 'NONE', #6036 ) ;
#20602=CARTESIAN_POINT ( 'NONE',  ( 100.0000000000000000, 269.9999999999999432, 145.0000000000000284 ) ) ;
#20608=CIRCLE ( 'NONE', #7070, 2.649999999999985700 ) ;
#20610=CARTESIAN_POINT ( 'NONE',  ( -100.0000000000000000, 269.9999999999999432, 145.0000000000000284 ) ) ;
#20627=EDGE_CURVE ( 'NONE', #14650, #16878, #11278, .T. ) ;
#20632=FACE_OUTER_BOUND ( 'NONE', #20852, .T. ) ;
#20640=CARTESIAN_POINT ( 'NONE',  ( 23.72315261474500048, -991.9446085409455236, 145.0000119999999697 ) ) ;
#20651=DIRECTION ( 'NONE',  ( 1.000000000000000000, 0.000000000000000000, 0.000000000000000000 ) ) ;
#20662=DIRECTION ( 'NONE',  ( 0.000000000000000000, 1.000000000000000000, 1.177509268541832635E-16 ) ) ;
#20669=CARTESIAN_POINT ( 'NONE',  ( -22.46865867768271841, -988.9158635398115393, -145.0000000000001137 ) ) ;
#20671=DIRECTION ( 'NONE',  ( 0.000000000000000000, 0.000000000000000000, -1.000000000000000000 ) ) ;
#20688=DIRECTION ( 'NONE',  ( 0.000000000000000000, 1.000000000000000000, 1.177509268541832635E-16 ) ) ;
#20694=CARTESIAN_POINT ( 'NONE',  ( -20.00000000000000000, 2.449293598294706513E-15, -150.0000000000000000 ) ) ;
#20710=LINE ( 'NONE', #7923, #14573 ) ;
#20725=DIRECTION ( 'NONE',  ( 0.000000000000000000, 0.000000000000000000, 1.000000000000000000 ) ) ;
#20737=ORIENTED_EDGE ( 'NONE', *, *, #23587, .T. ) ;
#20743=AXIS2_PLACEMENT_3D ( 'NONE', #15088, #17008, #22530 ) ;
#20744=VECTOR ( 'NONE', #16657, 1000.000000000000000 ) ;
#20750=ADVANCED_FACE ( 'NONE', ( #6170 ), #1179, .F. ) ;
#20751=ORIENTED_EDGE ( 'NONE', *, *, #6202, .T. ) ;
#20755=ORIENTED_EDGE ( 'NONE', *, *, #4332, .F. ) ;
#20769=VERTEX_POINT ( 'NONE', #1288 ) ;
#20790=ORIENTED_EDGE ( 'NONE', *, *, #16670, .T. ) ;
#20795=ADVANCED_FACE ( 'NONE', ( #5156 ), #16038, .F. ) ;
#20807=AXIS2_PLACEMENT_3D ( 'NONE', #22874, #9867, #6343 ) ;
#20815=CARTESIAN_POINT ( 'NONE',  ( 40.00000000000000000, 100.0000000000000000, 125.0000000000000000 ) ) ;
#20819=FACE_BOUND ( 'NONE', #21563, .T. ) ;
#20820=EDGE_LOOP ( 'NONE', ( #10893, #17638 ) ) ;
#20822=CYLINDRICAL_SURFACE ( 'NONE', #23421, 2.649999999999999467 ) ;
#20824=CARTESIAN_POINT ( 'NONE',  ( 0.000000000000000000, -1000.000000000000000, -125.0000000000001137 ) ) ;
#20833=LINE ( 'NONE', #7663, #11838 ) ;
#20840=CARTESIAN_POINT ( 'NONE',  ( 0.000000000000000000, 1.865214261513747767E-15, -138.9999999999999716 ) ) ;
#20848=CARTESIAN_POINT ( 'NONE',  ( -45.00000000000000000, 250.0000000000000000, -5.249999999999956479 ) ) ;
#20852=EDGE_LOOP ( 'NONE', ( #15839, #4682, #4378, #17626 ) ) ;
#20855=DIRECTION ( 'NONE',  ( 0.000000000000000000, 0.000000000000000000, 1.000000000000000000 ) ) ;
#20857=EDGE_CURVE ( 'NONE', #19306, #18285, #18093, .T. ) ;
#20863=CARTESIAN_POINT ( 'NONE',  ( 45.00000000000000000, 269.9999999999999432, 5.249999999999973355 ) ) ;
#20868=FACE_BOUND ( 'NONE', #3911, .T. ) ;
#20879=CARTESIAN_POINT ( 'NONE',  ( 24.20041621714725011, -6.482064212728088748, 145.0000119999999697 ) ) ;
#20906=ADVANCED_FACE ( 'NONE', ( #12681, #9382, #20116, #7436, #7553 ), #18297, .F. ) ;
#20917=LINE ( 'NONE', #22484, #19242 ) ;
#20925=DIRECTION ( 'NONE',  ( 0.000000000000000000, 1.000000000000000000, 0.000000000000000000 ) ) ;
#20937=LINE ( 'NONE', #777, #3 ) ;
#20945=B_SPLINE_CURVE_WITH_KNOTS ( 'NONE', 3,
 ( #13986, #17452, #21193, #8037, #4762, #6336, #11936, #9859, #19249, #17557, #13519, #4291, #17341, #6226, #1007, #13634, #4656, #13862, #15539, #12069, #20947, #7912, #21309, #791, #4403, #19364, #2467, #891, #11812, #8274, #2822, #8169, #22864, #13745 ),
 .UNSPECIFIED., .F., .F.,
 ( 4, 2, 2, 2, 2, 2, 2, 2, 2, 2, 2, 2, 2, 2, 2, 2, 4 ),
 ( 0.2500000000000000000, 0.2812500000000000000, 0.3125000000000000000, 0.3437500000000000000, 0.3750000000000000000, 0.4062500000000000000, 0.4375000000000000000, 0.4687500000000000000, 0.5000000000000000000, 0.5312500000000000000, 0.5625000000000000000, 0.5937500000000000000, 0.6250000000000000000, 0.6562500000000000000, 0.6875000000000000000, 0.7187500000000000000, 0.7500000000000000000 ),
 .UNSPECIFIED. ) ;
#20947=CARTESIAN_POINT ( 'NONE',  ( -8.050072859967690064, 23.72540897006225791, -145.0000000000000000 ) ) ;
#20967=FACE_OUTER_BOUND ( 'NONE', #20170, .T. ) ;
#20969=CIRCLE ( 'NONE', #22107, 5.249999999999949374 ) ;
#20977=CARTESIAN_POINT ( 'NONE',  ( 0.000000000000000000, -1000.000000000000000, 138.9999999999999716 ) ) ;
#20978=CARTESIAN_POINT ( 'NONE',  ( 45.00000000000000000, 269.9999999999999432, -5.249999999999973355 ) ) ;
#20998=ORIENTED_EDGE ( 'NONE', *, *, #21833, .F. ) ;
#20999=FACE_OUTER_BOUND ( 'NONE', #8940, .T. ) ;
#21001=VECTOR ( 'NONE', #22854, 1000.000000000000000 ) ;
#21006=LINE ( 'NONE', #10275, #14439 ) ;
#21010=VECTOR ( 'NONE', #5907, 1000.000000000000000 ) ;
#21018=DIRECTION ( 'NONE',  ( 0.000000000000000000, -1.000000000000000000, -1.110223024625156540E-16 ) ) ;
#21024=CARTESIAN_POINT ( 'NONE',  ( -6.487492490819623647, -24.19938668346784638, -145.0000000000000000 ) ) ;
#21055=DIRECTION ( 'NONE',  ( -0.000000000000000000, -0.000000000000000000, 1.000000000000000000 ) ) ;
#21067=CARTESIAN_POINT ( 'NONE',  ( 20.00000000000000000, -1000.000000000000000, -125.0000000000001137 ) ) ;
#21092=DIRECTION ( 'NONE',  ( 0.000000000000000000, -1.000000000000000000, 0.000000000000000000 ) ) ;
#21097=DIRECTION ( 'NONE',  ( -0.000000000000000000, 1.000000000000000000, 0.000000000000000000 ) ) ;
#21121=AXIS2_PLACEMENT_3D ( 'NONE', #22347, #3978, #9555 ) ;
#21137=CIRCLE ( 'NONE', #2232, 25.00000000000000000 ) ;
#21140=CARTESIAN_POINT ( 'NONE',  ( -22.46856765562321812, -11.08409875796190214, -145.0000000000000000 ) ) ;
#21155=CARTESIAN_POINT ( 'NONE',  ( -24.83992656739931704, -996.7332239287533184, -145.0000000000001421 ) ) ;
#21177=ORIENTED_EDGE ( 'NONE', *, *, #3202, .T. ) ;
#21190=CIRCLE ( 'NONE', #6914, 2.649999999999985700 ) ;
#21193=CARTESIAN_POINT ( 'NONE',  ( 24.84002319582486606, 3.266795291537505808, -145.0000000000000284 ) ) ;
#21201=CARTESIAN_POINT ( 'NONE',  ( 100.0000000000000000, 270.0000000000000000, -144.9999999999999716 ) ) ;
#21216=DIRECTION ( 'NONE',  ( 0.000000000000000000, 0.000000000000000000, 1.000000000000000000 ) ) ;
#21219=PLANE ( 'NONE',  #13475 ) ;
#21239=VERTEX_POINT ( 'NONE', #21201 ) ;
#21252=CARTESIAN_POINT ( 'NONE',  ( 100.0000000000000000, -1420.000000000000000, 124.9999999999998295 ) ) ;
#21259=EDGE_CURVE ( 'NONE', #13380, #7859, #21190, .T. ) ;
#21269=CARTESIAN_POINT ( 'NONE',  ( 3.266795293236424591, -24.84002319536234538, -145.0000000000000000 ) ) ;
#21309=CARTESIAN_POINT ( 'NONE',  ( -12.52399064354639613, 21.69904058266284608, -145.0000000000000000 ) ) ;
#21335=EDGE_LOOP ( 'NONE', ( #3703, #2763, #15628, #1656 ) ) ;
#21340=CARTESIAN_POINT ( 'NONE',  ( 12.52399064350059277, -1021.699040582693328, -145.0000000000001137 ) ) ;
#21345=ORIENTED_EDGE ( 'NONE', *, *, #18426, .T. ) ;
#21347=CARTESIAN_POINT ( 'NONE',  ( -67.34999999999996589, -87.33333333333338544, 145.0000000000000000 ) ) ;
#21359=FACE_OUTER_BOUND ( 'NONE', #8976, .T. ) ;
#21374=ORIENTED_EDGE ( 'NONE', *, *, #5116, .T. ) ;
#21380=EDGE_LOOP ( 'NONE', ( #15381, #6022 ) ) ;
#21384=ORIENTED_EDGE ( 'NONE', *, *, #16181, .F. ) ;
#21406=VERTEX_POINT ( 'NONE', #16824 ) ;
#21409=VERTEX_POINT ( 'NONE', #2082 ) ;
#21425=CIRCLE ( 'NONE', #3301, 5.249999999999949374 ) ;
#21433=VECTOR ( 'NONE', #23106, 1000.000000000000000 ) ;
#21434=ORIENTED_EDGE ( 'NONE', *, *, #2270, .T. ) ;
#21444=ADVANCED_FACE ( 'NONE', ( #8605 ), #23323, .F. ) ;
#21492=AXIS2_PLACEMENT_3D ( 'NONE', #20295, #5580, #3753 ) ;
#21505=FACE_OUTER_BOUND ( 'NONE', #13442, .T. ) ;
#21514=( NAMED_UNIT ( * ) PLANE_ANGLE_UNIT ( ) SI_UNIT ( $, .RADIAN. ) );
#21516=VERTEX_POINT ( 'NONE', #22957 ) ;
#21546=AXIS2_PLACEMENT_3D ( 'NONE', #13556, #15570, #11355 ) ;
#21563=EDGE_LOOP ( 'NONE', ( #17984, #21177 ) ) ;
#21577=VERTEX_POINT ( 'NONE', #4858 ) ;
#21583=FACE_OUTER_BOUND ( 'NONE', #16841, .T. ) ;
#21629=EDGE_CURVE ( 'NONE', #17037, #7464, #1811, .T. ) ;
#21638=VERTEX_POINT ( 'NONE', #3270 ) ;
#21669=DIRECTION ( 'NONE',  ( 0.000000000000000000, 1.000000000000000000, 0.000000000000000000 ) ) ;
#21680=CARTESIAN_POINT ( 'NONE',  ( 0.000000000000000000, 0.000000000000000000, -150.0000000000000000 ) ) ;
#21730=CARTESIAN_POINT ( 'NONE',  ( 24.99999999999998224, -1000.000000000000000, -145.0000060000000417 ) ) ;
#21746=FACE_OUTER_BOUND ( 'NONE', #11921, .T. ) ;
#21766=DIRECTION ( 'NONE',  ( 1.000000000000000000, 0.000000000000000000, 0.000000000000000000 ) ) ;
#21780=CARTESIAN_POINT ( 'NONE',  ( 67.35000000000002274, -112.6666666666666714, 124.9999999999999858 ) ) ;
#21784=LINE ( 'NONE', #16471, #22269 ) ;
#21787=AXIS2_PLACEMENT_3D ( 'NONE', #18211, #13052, #20132 ) ;
#21814=ORIENTED_EDGE ( 'NONE', *, *, #17835, .T. ) ;
#21833=EDGE_CURVE ( 'NONE', #19773, #20258, #19953, .T. ) ;
#21835=VERTEX_POINT ( 'NONE', #18617 ) ;
#21840=CARTESIAN_POINT ( 'NONE',  ( 11.07878015919985870, -22.47082401081930314, 145.0000119999999697 ) ) ;
#21844=CIRCLE ( 'NONE', #18765, 5.249999999999949374 ) ;
#21855=CARTESIAN_POINT ( 'NONE',  ( -24.20041621714723235, -1006.482064212727892, 145.0000119999999413 ) ) ;
#21861=DIRECTION ( 'NONE',  ( 0.000000000000000000, -1.110223024625156540E-16, 1.000000000000000000 ) ) ;
#21874=DIRECTION ( 'NONE',  ( 1.000000000000000000, 0.000000000000000000, 0.000000000000000000 ) ) ;
#21881=CIRCLE ( 'NONE', #3778, 24.99999999999998224 ) ;
#21883=LINE ( 'NONE', #16461, #22581 ) ;
#21884=ORIENTED_EDGE ( 'NONE', *, *, #4904, .F. ) ;
#21890=AXIS2_PLACEMENT_3D ( 'NONE', #13531, #8054, #22410 ) ;
#21895=CIRCLE ( 'NONE', #20743, 2.649999999999985700 ) ;
#21900=EDGE_CURVE ( 'NONE', #15535, #7773, #3352, .T. ) ;
#21904=LINE ( 'NONE', #5381, #3323 ) ;
#21923=CARTESIAN_POINT ( 'NONE',  ( -18.83467029480912203, 16.52066876451825550, 145.0000119999999697 ) ) ;
#21929=EDGE_CURVE ( 'NONE', #14713, #18285, #3104, .T. ) ;
#21938=EDGE_LOOP ( 'NONE', ( #2666, #17125 ) ) ;
#21965=B_SPLINE_CURVE_WITH_KNOTS ( 'NONE', 3,
 ( #13220, #9551, #385, #13327, #20640, #11646, #18950, #17158, #615, #7977, #11759, #17280, #7425, #7659, #11214, #5734, #13155, #9262, #2214, #2096, #16622, #16979, #11080, #22034, #20213, #5496, #18286, #20460, #11436, #16728, #22262, #20108, #11324, #13024 ),
 .UNSPECIFIED., .F., .F.,
 ( 4, 2, 2, 2, 2, 2, 2, 2, 2, 2, 2, 2, 2, 2, 2, 2, 4 ),
 ( 0.000000000000000000, 0.03125000000000000000, 0.06250000000000000000, 0.09375000000000000000, 0.1250000000000000000, 0.1562500000000000000, 0.1875000000000000000, 0.2187500000000000000, 0.2500000000000000000, 0.2812500000000000000, 0.3125000000000000000, 0.3437500000000000000, 0.3750000000000000000, 0.4062500000000000000, 0.4375000000000000000, 0.4687500000000000000, 0.5000000000000000000 ),
 .UNSPECIFIED. ) ;
#22016=CARTESIAN_POINT ( 'NONE',  ( 18.83879023463319058, -983.4833815101718528, -145.0000000000001421 ) ) ;
#22034=CARTESIAN_POINT ( 'NONE',  ( -15.24974479720505549, -980.1223093604608039, 145.0000119999999697 ) ) ;
#22035=ORIENTED_EDGE ( 'NONE', *, *, #2894, .F. ) ;
#22044=CARTESIAN_POINT ( 'NONE',  ( 23.72528575886166990, -1008.050112875828518, -145.0000000000001421 ) ) ;
#22067=VERTEX_POINT ( 'NONE', #5270 ) ;
#22075=CARTESIAN_POINT ( 'NONE',  ( -24.99999999999999645, -1.636246173744688726, 145.0000119999999697 ) ) ;
#22078=ORIENTED_EDGE ( 'NONE', *, *, #6506, .F. ) ;
#22087=CARTESIAN_POINT ( 'NONE',  ( 24.83884780301425366, -1003.272451888078649, 145.0000119999999697 ) ) ;
#22107=AXIS2_PLACEMENT_3D ( 'NONE', #9743, #446, #312 ) ;
#22142=ORIENTED_EDGE ( 'NONE', *, *, #4638, .F. ) ;
#22189=CARTESIAN_POINT ( 'NONE',  ( -15.24974479720505904, -19.87769063953886572, 145.0000119999999697 ) ) ;
#22206=ORIENTED_EDGE ( 'NONE', *, *, #3662, .T. ) ;
#22224=ORIENTED_EDGE ( 'NONE', *, *, #7106, .F. ) ;
#22254=VECTOR ( 'NONE', #1558, 1000.000000000000000 ) ;
#22257=CARTESIAN_POINT ( 'NONE',  ( -24.99999999999998224, -1000.000000000000000, 145.0000059999999280 ) ) ;
#22262=CARTESIAN_POINT ( 'NONE',  ( -24.20041621714723945, -993.5179357872719947, 145.0000119999999697 ) ) ;
#22269=VECTOR ( 'NONE', #11067, 1000.000000000000000 ) ;
#22332=CYLINDRICAL_SURFACE ( 'NONE', #13286, 5.249999999999973355 ) ;
#22336=VECTOR ( 'NONE', #15642, 1000.000000000000000 ) ;
#22347=CARTESIAN_POINT ( 'NONE',  ( 0.000000000000000000, 0.000000000000000000, -138.9999999999999716 ) ) ;
#22410=DIRECTION ( 'NONE',  ( 0.000000000000000000, 1.000000000000000000, 1.177509268541832635E-16 ) ) ;
#22454=CARTESIAN_POINT ( 'NONE',  ( 8.050072860899410543, -1023.725408969439172, -145.0000000000001137 ) ) ;
#22481=DIRECTION ( 'NONE',  ( 1.000000000000000000, 0.000000000000000000, 0.000000000000000000 ) ) ;
#22483=CARTESIAN_POINT ( 'NONE',  ( 6.487740029697272703, -975.8006625472378346, -145.0000000000001137 ) ) ;
#22484=CARTESIAN_POINT ( 'NONE',  ( -67.34999999999996589, -112.6666666666667140, 148.0000000000000000 ) ) ;
#22499=CARTESIAN_POINT ( 'NONE',  ( -69.99999999999997158, -87.33333333333338544, 145.0000000000000000 ) ) ;
#22529=EDGE_LOOP ( 'NONE', ( #14584, #16689, #19180, #16426 ) ) ;
#22530=DIRECTION ( 'NONE',  ( 0.000000000000000000, 1.000000000000000000, 0.000000000000000000 ) ) ;
#22531=DIRECTION ( 'NONE',  ( -0.000000000000000000, -0.000000000000000000, 1.000000000000000000 ) ) ;
#22538=LINE ( 'NONE', #342, #15598 ) ;
#22563=CARTESIAN_POINT ( 'NONE',  ( -69.99999999999997158, -112.6666666666667140, 124.9999999999999858 ) ) ;
#22570=CARTESIAN_POINT ( 'NONE',  ( -16.51654882469417984, -1018.838720569499060, -145.0000000000001421 ) ) ;
#22581=VECTOR ( 'NONE', #10939, 1000.000000000000000 ) ;
#22620=DIRECTION ( 'NONE',  ( 0.000000000000000000, 0.000000000000000000, 1.000000000000000000 ) ) ;
#22624=ORIENTED_EDGE ( 'NONE', *, *, #1472, .T. ) ;
#22640=EDGE_CURVE ( 'NONE', #7088, #2989, #18821, .T. ) ;
#22641=ORIENTED_EDGE ( 'NONE', *, *, #11867, .F. ) ;
#22658=CARTESIAN_POINT ( 'NONE',  ( 100.0000000000000000, -1400.000000000000000, 124.9999999999998295 ) ) ;
#22661=FACE_BOUND ( 'NONE', #21380, .T. ) ;
#22706=CARTESIAN_POINT ( 'NONE',  ( 0.000000000000000000, -1000.000000000000000, 124.9999999999998579 ) ) ;
#22710=( GEOMETRIC_REPRESENTATION_CONTEXT ( 3 ) GLOBAL_UNCERTAINTY_ASSIGNED_CONTEXT ( ( #4372 ) ) GLOBAL_UNIT_ASSIGNED_CONTEXT ( ( #12426, #10473, #4658 ) ) REPRESENTATION_CONTEXT ( 'NONE', 'WORKASPACE' ) );
#22711=CARTESIAN_POINT ( 'NONE',  ( -19.87444003266270087, -15.25452100728112015, -145.0000000000000000 ) ) ;
#22726=CARTESIAN_POINT ( 'NONE',  ( 20.00000000000000000, 0.000000000000000000, -138.9999999999999716 ) ) ;
#22732=VECTOR ( 'NONE', #6915, 1000.000000000000000 ) ;
#22758=CIRCLE ( 'NONE', #12403, 20.00000000000000000 ) ;
#22759=CIRCLE ( 'NONE', #14315, 25.00000000000000000 ) ;
#22773=CARTESIAN_POINT ( 'NONE',  ( -24.20041621714725721, 6.482064212728078090, 145.0000119999999697 ) ) ;
#22776=FACE_BOUND ( 'NONE', #20502, .T. ) ;
#22781=LINE ( 'NONE', #13180, #5329 ) ;
#22787=EDGE_CURVE ( 'NONE', #7773, #18735, #527, .T. ) ;
#22788=CARTESIAN_POINT ( 'NONE',  ( 70.00000000000000000, -112.6666666666666714, 148.0000000000000000 ) ) ;
#22800=ORIENTED_EDGE ( 'NONE', *, *, #13492, .T. ) ;
#22816=DIRECTION ( 'NONE',  ( 0.000000000000000000, 0.000000000000000000, 1.000000000000000000 ) ) ;
#22827=CARTESIAN_POINT ( 'NONE',  ( -24.84002319583889573, -3.266795291467043061, -145.0000000000000284 ) ) ;
#22837=CARTESIAN_POINT ( 'NONE',  ( -15.25452100747948769, -980.1255599675661188, -145.0000000000001421 ) ) ;
#22845=VERTEX_POINT ( 'NONE', #12841 ) ;
#22849=CARTESIAN_POINT ( 'NONE',  ( 72.64999999999999147, -112.6666666666666714, 148.0000000000000000 ) ) ;
#22851=ORIENTED_EDGE ( 'NONE', *, *, #4425, .T. ) ;
#22854=DIRECTION ( 'NONE',  ( 0.000000000000000000, 0.000000000000000000, 1.000000000000000000 ) ) ;
#22855=DIRECTION ( 'NONE',  ( 0.000000000000000000, 1.000000000000000000, 0.000000000000000000 ) ) ;
#22862=CARTESIAN_POINT ( 'NONE',  ( 0.000000000000000000, 0.000000000000000000, 138.9999999999999716 ) ) ;
#22864=CARTESIAN_POINT ( 'NONE',  ( -25.00004926069054889, 1.642023387880738872, -145.0000000000000000 ) ) ;
#22870=AXIS2_PLACEMENT_3D ( 'NONE', #23111, #6587, #4523 ) ;
#22874=CARTESIAN_POINT ( 'NONE',  ( 40.00000000000000000, 100.0000000000000000, 150.2000000000009550 ) ) ;
#22877=VERTEX_POINT ( 'NONE', #21730 ) ;
#22935=EDGE_CURVE ( 'NONE', #13307, #3094, #13069, .T. ) ;
#22938=CARTESIAN_POINT ( 'NONE',  ( -24.19924082432261869, -6.487720809339531769, -144.9999999999999716 ) ) ;
#22939=VERTEX_POINT ( 'NONE', #7718 ) ;
#22957=CARTESIAN_POINT ( 'NONE',  ( 100.0000000000000000, 269.9999999999999432, 145.0000000000000284 ) ) ;
#22993=CARTESIAN_POINT ( 'NONE',  ( 0.000000000000000000, -1000.000000000000000, -138.9999999999999716 ) ) ;
#23001=ORIENTED_EDGE ( 'NONE', *, *, #13168, .F. ) ;
#23015=DIRECTION ( 'NONE',  ( 1.000000000000000000, 0.000000000000000000, 0.000000000000000000 ) ) ;
#23016=CARTESIAN_POINT ( 'NONE',  ( -45.00000000000000000, 272.9999999999999432, -5.249999999999973355 ) ) ;
#23029=CARTESIAN_POINT ( 'NONE',  ( 0.000000000000000000, 1.865214261513747767E-15, 145.0000119999999697 ) ) ;
#23039=ADVANCED_FACE ( 'NONE', ( #12950 ), #3711, .F. ) ;
#23059=CARTESIAN_POINT ( 'NONE',  ( -16.51654882469418695, -18.83872056949901008, -145.0000000000000000 ) ) ;
#23098=CARTESIAN_POINT ( 'NONE',  ( -20.00000000000000000, -1000.000000000000000, 138.9999999999999716 ) ) ;
#23106=DIRECTION ( 'NONE',  ( 0.000000000000000000, 0.000000000000000000, -1.000000000000000000 ) ) ;
#23109=ORIENTED_EDGE ( 'NONE', *, *, #7800, .T. ) ;
#23111=CARTESIAN_POINT ( 'NONE',  ( 40.00000000000000000, 100.0000000000000000, 145.0000000000000000 ) ) ;
#23129=DIRECTION ( 'NONE',  ( -1.000000000000000000, 0.000000000000000000, 0.000000000000000000 ) ) ;
#23151=CARTESIAN_POINT ( 'NONE',  ( 1.641270926519074358, -1025.000000000000000, -145.0000000000001421 ) ) ;
#23160=EDGE_LOOP ( 'NONE', ( #5938, #17850, #1668, #665 ) ) ;
#23191=CARTESIAN_POINT ( 'NONE',  ( -12.52400585386708443, -21.69891193169445032, -145.0000000000000000 ) ) ;
#23218=ORIENTED_EDGE ( 'NONE', *, *, #18935, .F. ) ;
#23238=DIRECTION ( 'NONE',  ( 0.000000000000000000, 1.000000000000000000, 0.000000000000000000 ) ) ;
#23243=DIRECTION ( 'NONE',  ( 1.000000000000000000, 0.000000000000000000, 0.000000000000000000 ) ) ;
#23249=DIRECTION ( 'NONE',  ( 0.000000000000000000, -1.177509268541832635E-16, 1.000000000000000000 ) ) ;
#23258=CARTESIAN_POINT ( 'NONE',  ( 18.83872056894873381, -1016.516548825274981, -145.0000000000001421 ) ) ;
#23304=AXIS2_PLACEMENT_3D ( 'NONE', #12295, #19602, #58 ) ;
#23323=CYLINDRICAL_SURFACE ( 'NONE', #2263, 5.249999999999942268 ) ;
#23330=CARTESIAN_POINT ( 'NONE',  ( 100.0000000000000000, 250.0000000000000000, -124.9999999999999716 ) ) ;
#23337=ORIENTED_EDGE ( 'NONE', *, *, #9723, .T. ) ;
#23366=FACE_OUTER_BOUND ( 'NONE', #16319, .T. ) ;
#23371=CIRCLE ( 'NONE', #13007, 24.99999999999998224 ) ;
#23382=VERTEX_POINT ( 'NONE', #10979 ) ;
#23383=PLANE ( 'NONE',  #20045 ) ;
#23385=ADVANCED_FACE ( 'NONE', ( #1872 ), #14580, .F. ) ;
#23417=EDGE_LOOP ( 'NONE', ( #17667, #7038, #5972, #15809 ) ) ;
#23421=AXIS2_PLACEMENT_3D ( 'NONE', #9967, #9846, #654 ) ;
#23460=LINE ( 'NONE', #9345, #10805 ) ;
#23491=CYLINDRICAL_SURFACE ( 'NONE', #15693, 20.00000000000000000 ) ;
#23517=CARTESIAN_POINT ( 'NONE',  ( 18.83467029480910426, 16.52066876451826971, 145.0000119999999697 ) ) ;
#23525=VECTOR ( 'NONE', #23683, 1000.000000000000000 ) ;
#23558=CARTESIAN_POINT ( 'NONE',  ( 25.00004926069054889, -1.642023387880738872, -145.0000000000000000 ) ) ;
#23573=ORIENTED_EDGE ( 'NONE', *, *, #4181, .F. ) ;
#23574=ORIENTED_EDGE ( 'NONE', *, *, #17560, .F. ) ;
#23587=EDGE_CURVE ( 'NONE', #13361, #14650, #2674, .T. ) ;
#23607=ADVANCED_FACE ( 'NONE', ( #17100 ), #15659, .F. ) ;
#23611=EDGE_LOOP ( 'NONE', ( #16176, #19423 ) ) ;
#23624=DIRECTION ( 'NONE',  ( 0.000000000000000000, -1.000000000000000000, 0.000000000000000000 ) ) ;
#23632=ORIENTED_EDGE ( 'NONE', *, *, #2683, .T. ) ;
#23652=ADVANCED_FACE ( 'NONE', ( #7801 ), #798, .F. ) ;
#23667=CIRCLE ( 'NONE', #10194, 5.249999999999956479 ) ;
#23683=DIRECTION ( 'NONE',  ( -0.000000000000000000, 1.000000000000000000, -0.000000000000000000 ) ) ;
#23687=CARTESIAN_POINT ( 'NONE',  ( 0.000000000000000000, -1000.000000000000000, -138.9999999999999716 ) ) ;
#23696=AXIS2_PLACEMENT_3D ( 'NONE', #9792, #5810, #16904 ) ;
#23705=DIRECTION ( 'NONE',  ( 0.000000000000000000, -1.177509268541832635E-16, 1.000000000000000000 ) ) ;
#23716=DIRECTION ( 'NONE',  ( 1.000000000000000000, 0.000000000000000000, 0.000000000000000000 ) ) ;
#23767=ORIENTED_EDGE ( 'NONE', *, *, #6506, .T. ) ;
#23783=CYLINDRICAL_SURFACE ( 'NONE', #7906, 20.00000000000000000 ) ;
#23787=CARTESIAN_POINT ( 'NONE',  ( -18.83467029480908295, -1016.520668764518291, 145.0000119999999697 ) ) ;
#23928=COLOUR_RGB('Off White',0.89,0.88,0.83);
#23929=FILL_AREA_STYLE_COLOUR('',#23928);
#23930=FILL_AREA_STYLE('',(#23929));
#23931=SURFACE_STYLE_FILL_AREA(#23930);
#23932=SURFACE_SIDE_STYLE('',(#23931));
#23933=SURFACE_STYLE_USAGE(.BOTH.,#23932);
#23934=PRESENTATION_STYLE_ASSIGNMENT((#23933));
ENDSEC;
END-ISO-10303-21;
